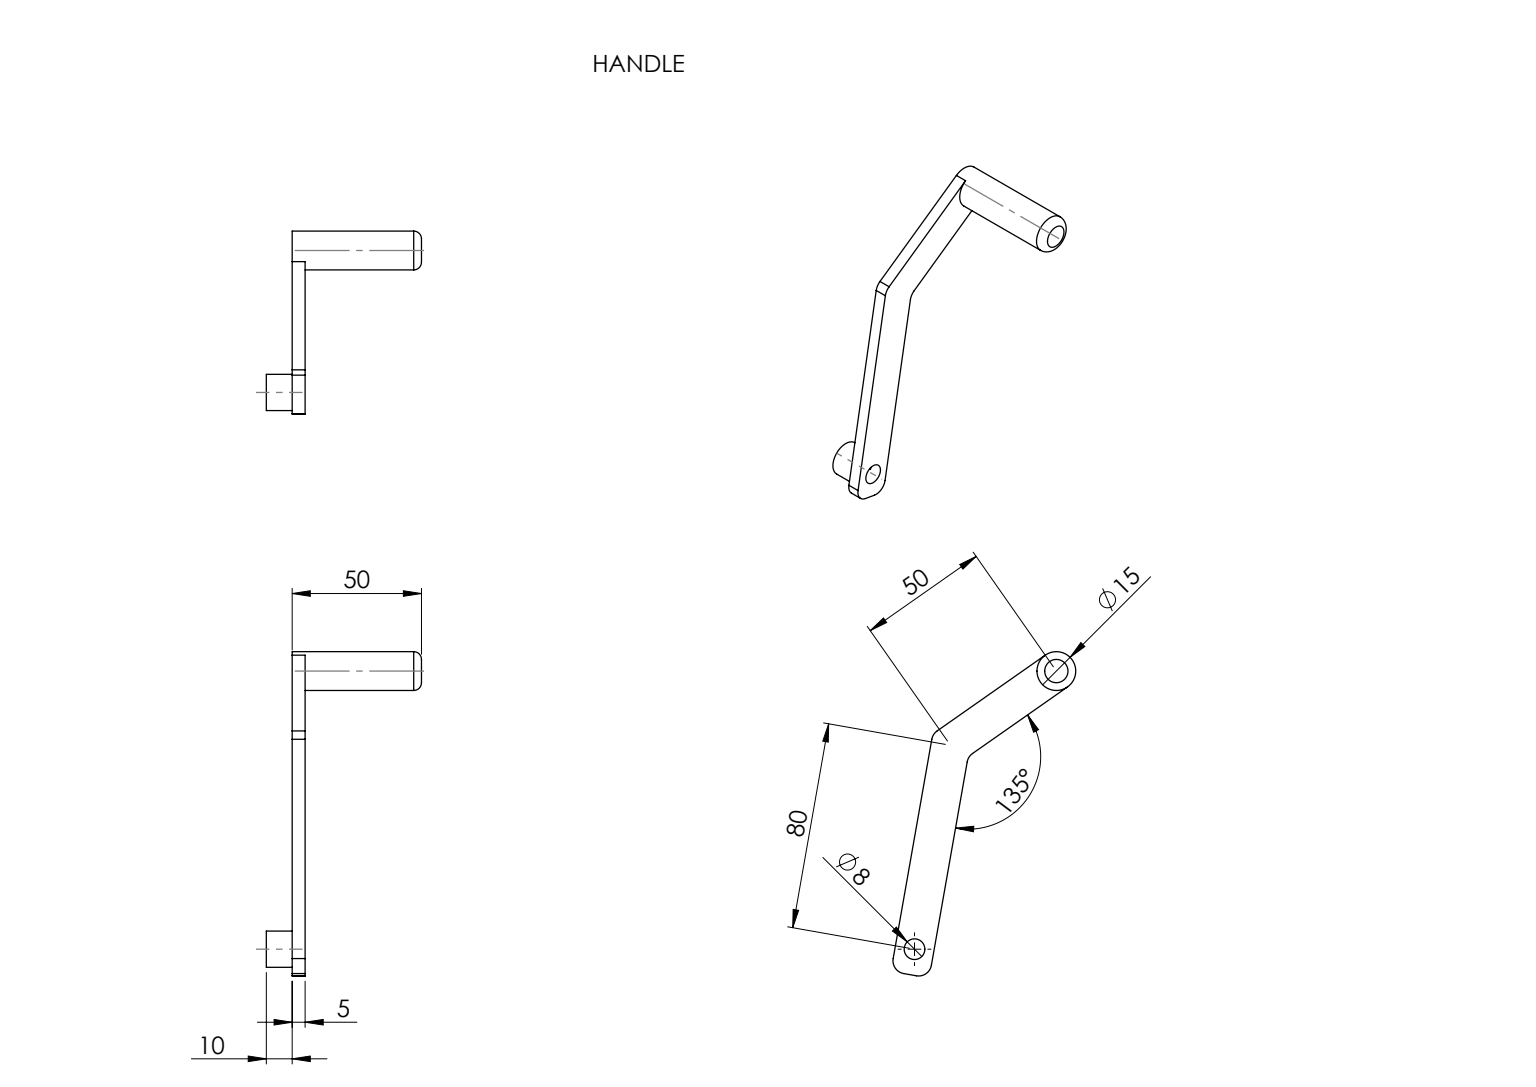
ISO-10303-21;
HEADER;
FILE_DESCRIPTION (('STEP AP214'),
    '1' );
FILE_NAME ('handle.step',
    '2026-09-28T15:49:00',
    ( '' ),
    ( '' ),
    'SwSTEP 2.0',
    'SolidWorks 2026',
    '' );
FILE_SCHEMA (( 'AUTOMOTIVE_DESIGN' ));
ENDSEC;

DATA;
#56=CARTESIAN_POINT ( 'NONE',  ( 55.00000000000000711, -25.98076211353320986, 88.99999999999994316 ) ) ;
#130=ORIENTED_EDGE ( 'NONE', *, *, #26286, .T. ) ;
#133=ORIENTED_EDGE ( 'NONE', *, *, #25065, .T. ) ;
#143=EDGE_CURVE ( 'NONE', #14032, #9695, #27885, .T. ) ;
#156=CARTESIAN_POINT ( 'NONE',  ( 65.00000000000001421, 81.48267994499606459, 30.15054357219658954 ) ) ;
#190=ADVANCED_FACE ( 'NONE', ( #12334 ), #23311, .F. ) ;
#261=AXIS2_PLACEMENT_3D ( 'NONE', #4805, #2292, #35227 ) ;
#346=FILL_AREA_STYLE ('',( #33832 ) ) ;
#366=DIRECTION ( 'NONE',  ( -1.000000000000000000, 0.000000000000000000, 0.000000000000000000 ) ) ;
#383=EDGE_CURVE ( 'NONE', #18596, #21774, #10521, .T. ) ;
#428=VERTEX_POINT ( 'NONE', #27465 ) ;
#447=VECTOR ( 'NONE', #3446, 1000.000000000000000 ) ;
#515=DIRECTION ( 'NONE',  ( 0.000000000000000000, 0.000000000000000000, 1.000000000000000000 ) ) ;
#636=CARTESIAN_POINT ( 'NONE',  ( 70.00000000000001421, -37.13120097615721704, 79.35042362907756797 ) ) ;
#776=CARTESIAN_POINT ( 'NONE',  ( 70.00000000000001421, 87.62632027716348659, 34.45236684482946288 ) ) ;
#781=CARTESIAN_POINT ( 'NONE',  ( 70.00000000000001421, 45.53424681125909501, 59.69714175238111409 ) ) ;
#809=FACE_OUTER_BOUND ( 'NONE', #28343, .T. ) ;
#841=AXIS2_PLACEMENT_3D ( 'NONE', #19896, #5545, #8749 ) ;
#904=EDGE_CURVE ( 'NONE', #3203, #33824, #4242, .T. ) ;
#982=CARTESIAN_POINT ( 'NONE',  ( 65.00000000000001421, -25.98076211353320986, 84.99999999999994316 ) ) ;
#1054=CARTESIAN_POINT ( 'NONE',  ( 70.00000000000001421, -30.47068043442695284, 88.33026027086506815 ) ) ;
#1165=SURFACE_STYLE_FILL_AREA ( #31929 ) ;
#1182=FACE_OUTER_BOUND ( 'NONE', #21588, .T. ) ;
#1194=LINE ( 'NONE', #23141, #2335 ) ;
#1235=CARTESIAN_POINT ( 'NONE',  ( 65.00000000000001421, -25.98076211353320986, 84.99999999999994316 ) ) ;
#1255=DIRECTION ( 'NONE',  ( 1.000000000000000000, -0.000000000000000000, -0.000000000000000000 ) ) ;
#1269=EDGE_LOOP ( 'NONE', ( #4591, #17269, #21862, #33608, #20840, #6158, #6470, #4785 ) ) ;
#1271=ORIENTED_EDGE ( 'NONE', *, *, #26959, .F. ) ;
#1314=DIRECTION ( 'NONE',  ( 0.000000000000000000, -8.326672684688666165E-15, 1.000000000000000000 ) ) ;
#1354=DIRECTION ( 'NONE',  ( 0.000000000000000000, -0.1736481776669211718, -0.9848077530122096857 ) ) ;
#1451=CIRCLE ( 'NONE', #16950, 7.499999999999992895 ) ;
#1492=ORIENTED_EDGE ( 'NONE', *, *, #25065, .F. ) ;
#1496=ORIENTED_EDGE ( 'NONE', *, *, #16220, .F. ) ;
#1573=CARTESIAN_POINT ( 'NONE',  ( 70.00001200000002655, -29.87665282020647695, 83.95300846256282057 ) ) ;
#1611=TOROIDAL_SURFACE ( 'NONE', #5092, 4.499999999999990230, 3.000000000000000000 ) ;
#1670=LINE ( 'NONE', #12654, #13772 ) ;
#1760=CARTESIAN_POINT ( 'NONE',  ( 55.00000000000000711, -26.94801722181409431, 85.25380613764163229 ) ) ;
#1767=LINE ( 'NONE', #20817, #16991 ) ;
#1817=PLANE ( 'NONE',  #32446 ) ;
#1843=EDGE_CURVE ( 'NONE', #25616, #5216, #33585, .T. ) ;
#1888=( NAMED_UNIT ( * ) PLANE_ANGLE_UNIT ( ) SI_UNIT ( $, .RADIAN. ) );
#1954=VERTEX_POINT ( 'NONE', #21205 ) ;
#1975=AXIS2_PLACEMENT_3D ( 'NONE', #6813, #4502, #17962 ) ;
#2064=ADVANCED_FACE ( 'NONE', ( #14500 ), #4316, .T. ) ;
#2150=DIRECTION ( 'NONE',  ( -1.000000000000000000, 0.000000000000000000, 0.000000000000000000 ) ) ;
#2194=ORIENTED_EDGE ( 'NONE', *, *, #3621, .F. ) ;
#2216=ORIENTED_EDGE ( 'NONE', *, *, #904, .F. ) ;
#2232=PLANE ( 'NONE',  #16375 ) ;
#2253=VECTOR ( 'NONE', #6220, 1000.000000000000114 ) ;
#2276=DIRECTION ( 'NONE',  ( 0.000000000000000000, 0.000000000000000000, 1.000000000000000000 ) ) ;
#2292=DIRECTION ( 'NONE',  ( -1.000000000000000000, -0.000000000000000000, -0.000000000000000000 ) ) ;
#2335=VECTOR ( 'NONE', #23318, 999.9999999999998863 ) ;
#2380=CARTESIAN_POINT ( 'NONE',  ( 70.00001200000004076, -24.93377057609608372, 88.89589070667321380 ) ) ;
#2403=DIRECTION ( 'NONE',  ( 0.000000000000000000, -2.775557561562888984E-15, 1.000000000000000000 ) ) ;
#2413=CARTESIAN_POINT ( 'NONE',  ( 65.00000000000001421, -25.98076211353320986, 88.99999999999994316 ) ) ;
#2450=ADVANCED_FACE ( 'NONE', ( #15932 ), #18461, .T. ) ;
#2497=CARTESIAN_POINT ( 'NONE',  ( 70.00000000000001421, -29.60243954609234507, 93.25429903592612391 ) ) ;
#2565=VERTEX_POINT ( 'NONE', #27993 ) ;
#2569=CARTESIAN_POINT ( 'NONE',  ( 65.00000000000001421, 75.33903961282865680, 25.84872029956372330 ) ) ;
#2593=ORIENTED_EDGE ( 'NONE', *, *, #13307, .T. ) ;
#2628=LINE ( 'NONE', #10536, #17242 ) ;
#2636=CYLINDRICAL_SURFACE ( 'NONE', #35102, 5.000000000000004441 ) ;
#2663=EDGE_CURVE ( 'NONE', #3203, #18596, #9362, .T. ) ;
#2735=DIRECTION ( 'NONE',  ( 0.000000000000000000, 0.000000000000000000, -1.000000000000000000 ) ) ;
#2741=AXIS2_PLACEMENT_3D ( 'NONE', #19253, #30776, #2735 ) ;
#2745=ORIENTED_EDGE ( 'NONE', *, *, #4160, .F. ) ;
#2809=CARTESIAN_POINT ( 'NONE',  ( 65.00000000000001421, 87.62632027716348659, 34.45236684482946288 ) ) ;
#2854=VERTEX_POINT ( 'NONE', #6203 ) ;
#2954=EDGE_CURVE ( 'NONE', #9823, #7205, #23657, .T. ) ;
#3203=VERTEX_POINT ( 'NONE', #10117 ) ;
#3222=CARTESIAN_POINT ( 'NONE',  ( 65.00000000000001421, -30.47068043442695284, 88.33026027086506815 ) ) ;
#3229=CARTESIAN_POINT ( 'NONE',  ( 65.00000000000001421, -32.20716221109618260, 78.48218274074299927 ) ) ;
#3232=AXIS2_PLACEMENT_3D ( 'NONE', #781, #25461, #19843 ) ;
#3269=DIRECTION ( 'NONE',  ( 0.000000000000000000, 0.2538061376417697357, 0.9672551082808334977 ) ) ;
#3276=ORIENTED_EDGE ( 'NONE', *, *, #9282, .T. ) ;
#3368=DIRECTION ( 'NONE',  ( 0.000000000000000000, 0.000000000000000000, 1.000000000000000000 ) ) ;
#3388=ORIENTED_EDGE ( 'NONE', *, *, #16220, .T. ) ;
#3389=EDGE_CURVE ( 'NONE', #2565, #13276, #17096, .T. ) ;
#3416=EDGE_CURVE ( 'NONE', #33336, #30332, #7608, .T. ) ;
#3446=DIRECTION ( 'NONE',  ( 1.000000000000000000, -0.000000000000000000, -0.000000000000000000 ) ) ;
#3489=CARTESIAN_POINT ( 'NONE',  ( 65.00000000000001421, -25.98076211353320986, 80.99999999999992895 ) ) ;
#3511=DIRECTION ( 'NONE',  ( 0.000000000000000000, 0.000000000000000000, 1.000000000000000000 ) ) ;
#3621=EDGE_CURVE ( 'NONE', #4878, #28758, #31678, .T. ) ;
#3638=ORIENTED_EDGE ( 'NONE', *, *, #5358, .T. ) ;
#3683=CARTESIAN_POINT ( 'NONE',  ( 70.00000000000001421, 0.000000000000000000, 0.000000000000000000 ) ) ;
#3724=ORIENTED_EDGE ( 'NONE', *, *, #24002, .T. ) ;
#3746=CIRCLE ( 'NONE', #17524, 5.000000000000004441 ) ;
#3769=CLOSED_SHELL ( 'NONE', ( #18687, #5338, #22527, #33299, #32877, #34808, #14774, #29471, #2450, #190, #15138, #32497, #4472, #4930, #4111, #33091, #6476, #7953, #7065, #31290, #10902, #2064, #24425, #21358, #22284, #3966 ) ) ;
#3787=ORIENTED_EDGE ( 'NONE', *, *, #14974, .T. ) ;
#3796=CARTESIAN_POINT ( 'NONE',  ( 112.0000000000000000, 81.48267994499606459, 37.65054357219658243 ) ) ;
#3860=CARTESIAN_POINT ( 'NONE',  ( 70.00000000000001421, -30.47068043442695284, 93.33026027086508236 ) ) ;
#3893=PLANE ( 'NONE',  #22062 ) ;
#3910=VECTOR ( 'NONE', #4653, 999.9999999999998863 ) ;
#3932=CARTESIAN_POINT ( 'NONE',  ( 70.00001200000002655, -29.17942948312593998, 82.54181312010028648 ) ) ;
#3966=ADVANCED_FACE ( 'NONE', ( #5911 ), #17055, .F. ) ;
#3993=EDGE_CURVE ( 'NONE', #20175, #14032, #8812, .T. ) ;
#4111=ADVANCED_FACE ( 'NONE', ( #25901, #17767 ), #23356, .T. ) ;
#4136=( NAMED_UNIT ( * ) SI_UNIT ( $, .STERADIAN. ) SOLID_ANGLE_UNIT ( ) );
#4160=EDGE_CURVE ( 'NONE', #34443, #26484, #18590, .T. ) ;
#4235=ORIENTED_EDGE ( 'NONE', *, *, #8593, .T. ) ;
#4241=DIRECTION ( 'NONE',  ( 0.000000000000000000, 0.000000000000000000, 1.000000000000000000 ) ) ;
#4242=CIRCLE ( 'NONE', #30675, 4.499999999999990230 ) ;
#4271=EDGE_CURVE ( 'NONE', #2854, #9753, #31822, .T. ) ;
#4316=TOROIDAL_SURFACE ( 'NONE', #841, 4.499999999999990230, 3.000000000000000000 ) ;
#4373=ORIENTED_EDGE ( 'NONE', *, *, #3621, .T. ) ;
#4472=ADVANCED_FACE ( 'NONE', ( #809 ), #3893, .T. ) ;
#4502=DIRECTION ( 'NONE',  ( -1.000000000000000000, 0.000000000000000000, 0.000000000000000000 ) ) ;
#4503=ORIENTED_EDGE ( 'NONE', *, *, #17218, .F. ) ;
#4521=STYLED_ITEM ( 'NONE', ( #15434 ), #33750 ) ;
#4547=SHAPE_REPRESENTATION ( 'handle', ( #21307 ), #23057 ) ;
#4565=ORIENTED_EDGE ( 'NONE', *, *, #18024, .T. ) ;
#4591=ORIENTED_EDGE ( 'NONE', *, *, #12276, .T. ) ;
#4592=ORIENTED_EDGE ( 'NONE', *, *, #3389, .T. ) ;
#4617=DIRECTION ( 'NONE',  ( -0.000000000000000000, 0.8191520442889889120, 0.5735764363510502672 ) ) ;
#4632=ORIENTED_EDGE ( 'NONE', *, *, #7310, .T. ) ;
#4653=DIRECTION ( 'NONE',  ( 0.000000000000000000, 0.5735764363510502672, -0.8191520442889889120 ) ) ;
#4693=CYLINDRICAL_SURFACE ( 'NONE', #5183, 4.000000000000003553 ) ;
#4695=MECHANICAL_DESIGN_GEOMETRIC_PRESENTATION_REPRESENTATION('',(#10435),#28238);
#4730=CARTESIAN_POINT ( 'NONE',  ( 70.00000600000001327, -25.98076211353320986, 88.99999999999994316 ) ) ;
#4785=ORIENTED_EDGE ( 'NONE', *, *, #14974, .F. ) ;
#4805=CARTESIAN_POINT ( 'NONE',  ( 65.00000000000001421, -25.98076211353320986, 84.99999999999994316 ) ) ;
#4816=ORIENTED_EDGE ( 'NONE', *, *, #1843, .T. ) ;
#4878=VERTEX_POINT ( 'NONE', #31685 ) ;
#4930=ADVANCED_FACE ( 'NONE', ( #14936 ), #1817, .F. ) ;
#4995=FACE_OUTER_BOUND ( 'NONE', #23443, .T. ) ;
#5038=DIRECTION ( 'NONE',  ( 1.000000000000000000, -0.000000000000000000, -0.000000000000000000 ) ) ;
#5075=CARTESIAN_POINT ( 'NONE',  ( 65.00000000000001421, -30.47068043442695284, 93.33026027086508236 ) ) ;
#5076=VERTEX_POINT ( 'NONE', #32578 ) ;
#5078=CARTESIAN_POINT ( 'NONE',  ( 70.00001200000002655, -22.78209474394049039, 87.45818687989959983 ) ) ;
#5092=AXIS2_PLACEMENT_3D ( 'NONE', #30970, #366, #22858 ) ;
#5114=DIRECTION ( 'NONE',  ( -1.000000000000000000, -0.000000000000000000, -0.000000000000000000 ) ) ;
#5183=AXIS2_PLACEMENT_3D ( 'NONE', #18695, #7891, #21221 ) ;
#5209=EDGE_LOOP ( 'NONE', ( #23961, #2216, #35094, #7402 ) ) ;
#5216=VERTEX_POINT ( 'NONE', #33292 ) ;
#5272=CARTESIAN_POINT ( 'NONE',  ( 65.00000000000001421, -30.47068043442695284, 88.33026027086506815 ) ) ;
#5338=ADVANCED_FACE ( 'NONE', ( #22118 ), #5580, .T. ) ;
#5358=EDGE_CURVE ( 'NONE', #9823, #30224, #18658, .T. ) ;
#5379=AXIS2_PLACEMENT_3D ( 'NONE', #24595, #35586, #16814 ) ;
#5388=CARTESIAN_POINT ( 'NONE',  ( 55.00000000000000711, -25.99649394950422021, 81.00003093645240426 ) ) ;
#5395=AXIS2_PLACEMENT_3D ( 'NONE', #13673, #8252, #25002 ) ;
#5424=ORIENTED_EDGE ( 'NONE', *, *, #18024, .F. ) ;
#5445=DIRECTION ( 'NONE',  ( 1.000000000000000000, -0.000000000000000000, -0.000000000000000000 ) ) ;
#5473=PLANE ( 'NONE',  #10506 ) ;
#5484=ORIENTED_EDGE ( 'NONE', *, *, #20613, .F. ) ;
#5509=AXIS2_PLACEMENT_3D ( 'NONE', #21410, #7726, #18709 ) ;
#5515=EDGE_LOOP ( 'NONE', ( #12905, #15381 ) ) ;
#5545=DIRECTION ( 'NONE',  ( -1.000000000000000000, 0.000000000000000000, 0.000000000000000000 ) ) ;
#5580=CYLINDRICAL_SURFACE ( 'NONE', #27312, 7.499999999999992895 ) ;
#5598=DIRECTION ( 'NONE',  ( -1.000000000000000000, 0.000000000000000000, 0.000000000000000000 ) ) ;
#5723=EDGE_CURVE ( 'NONE', #25950, #34599, #1451, .T. ) ;
#5787=CARTESIAN_POINT ( 'NONE',  ( 55.00000000000000711, -25.98076211353320986, 84.99999999999994316 ) ) ;
#5849=ORIENTED_EDGE ( 'NONE', *, *, #14083, .T. ) ;
#5911=FACE_OUTER_BOUND ( 'NONE', #7615, .T. ) ;
#5954=LINE ( 'NONE', #25404, #447 ) ;
#5971=ORIENTED_EDGE ( 'NONE', *, *, #4271, .F. ) ;
#6022=ORIENTED_EDGE ( 'NONE', *, *, #14553, .F. ) ;
#6025=CARTESIAN_POINT ( 'NONE',  ( 55.00000000000000711, -25.98076211353320986, 80.99999999999992895 ) ) ;
#6145=ORIENTED_EDGE ( 'NONE', *, *, #14083, .F. ) ;
#6148=VECTOR ( 'NONE', #16787, 1000.000000000000000 ) ;
#6158=ORIENTED_EDGE ( 'NONE', *, *, #10194, .T. ) ;
#6159=ORIENTED_EDGE ( 'NONE', *, *, #3389, .F. ) ;
#6192=DIRECTION ( 'NONE',  ( -1.000000000000000000, 0.000000000000000000, 0.000000000000000000 ) ) ;
#6203=CARTESIAN_POINT ( 'NONE',  ( 65.00000000000001421, 49.63000703270403591, 62.56502393413636298 ) ) ;
#6220=DIRECTION ( 'NONE',  ( 0.000000000000000000, -0.2538061376417682924, -0.9672551082808338307 ) ) ;
#6295=ORIENTED_EDGE ( 'NONE', *, *, #26286, .F. ) ;
#6385=COLOUR_RGB ( '', 0.08235294, 0.09019608, 0.10196078) ;
#6409=AXIS2_PLACEMENT_3D ( 'NONE', #7493, #29294, #29648 ) ;
#6470=ORIENTED_EDGE ( 'NONE', *, *, #15880, .F. ) ;
#6472=CARTESIAN_POINT ( 'NONE',  ( 70.00000000000001421, -24.67840078103129997, 92.38605814759151258 ) ) ;
#6476=ADVANCED_FACE ( 'NONE', ( #28695 ), #28867, .F. ) ;
#6496=VECTOR ( 'NONE', #6192, 1000.000000000000000 ) ;
#6530=DIRECTION ( 'NONE',  ( -1.000000000000000000, -0.000000000000000000, -0.000000000000000000 ) ) ;
#6553=CARTESIAN_POINT ( 'NONE',  ( 70.00000000000001421, 58.35354061212520804, 76.25822877525452270 ) ) ;
#6707=CARTESIAN_POINT ( 'NONE',  ( 112.0000000000000000, 81.48267994499606459, 22.65054357219659664 ) ) ;
#6723=DIRECTION ( 'NONE',  ( -1.000000000000000000, 0.000000000000000000, 0.000000000000000000 ) ) ;
#6813=CARTESIAN_POINT ( 'NONE',  ( 70.00000000000001421, 45.53424681125909501, 59.69714175238111409 ) ) ;
#6927=DIRECTION ( 'NONE',  ( 0.000000000000000000, 0.9672551082808338307, -0.2538061376417690695 ) ) ;
#6962=CARTESIAN_POINT ( 'NONE',  ( 70.00001200000002655, -27.02775365097034310, 88.89589070667321380 ) ) ;
#6974=AXIS2_PLACEMENT_3D ( 'NONE', #21555, #34927, #10253 ) ;
#7016=DIRECTION ( 'NONE',  ( -0.000000000000000000, 0.2538061376417689585, 0.9672551082808338307 ) ) ;
#7063=VECTOR ( 'NONE', #16180, 1000.000000000000114 ) ;
#7065=ADVANCED_FACE ( 'NONE', ( #24276 ), #18186, .T. ) ;
#7102=CARTESIAN_POINT ( 'NONE',  ( 63.00000000000001421, -26.94801722181409431, 85.25380613764163229 ) ) ;
#7166=( LENGTH_UNIT ( ) NAMED_UNIT ( * ) SI_UNIT ( .MILLI., .METRE. ) );
#7205=VERTEX_POINT ( 'NONE', #21910 ) ;
#7282=DIRECTION ( 'NONE',  ( 0.000000000000000000, 0.2538061376417690140, 0.9672551082808337197 ) ) ;
#7310=EDGE_CURVE ( 'NONE', #428, #2565, #16848, .T. ) ;
#7388=ORIENTED_EDGE ( 'NONE', *, *, #28035, .F. ) ;
#7402=ORIENTED_EDGE ( 'NONE', *, *, #31805, .F. ) ;
#7466=CARTESIAN_POINT ( 'NONE',  ( 115.0000000000000000, 81.48267994499606459, 37.65054357219658243 ) ) ;
#7484=ORIENTED_EDGE ( 'NONE', *, *, #24002, .F. ) ;
#7493=CARTESIAN_POINT ( 'NONE',  ( 112.0000000000000000, 81.48267994499606459, 30.15054357219658954 ) ) ;
#7563=CARTESIAN_POINT ( 'NONE',  ( 70.00000000000001421, -35.39471919948800149, 89.19850115919967948 ) ) ;
#7576=CARTESIAN_POINT ( 'NONE',  ( 70.00001200000001234, -25.45716333793490449, 88.99999999999995737 ) ) ;
#7608=CIRCLE ( 'NONE', #27751, 4.000000000000003553 ) ;
#7615=EDGE_LOOP ( 'NONE', ( #33702, #6159, #32414, #32946 ) ) ;
#7645=CARTESIAN_POINT ( 'NONE',  ( 55.00000000000000711, -25.98076211353320986, 91.99999999999994316 ) ) ;
#7662=AXIS2_PLACEMENT_3D ( 'NONE', #1054, #12025, #28593 ) ;
#7714=EDGE_CURVE ( 'NONE', #28924, #33336, #16617, .T. ) ;
#7726=DIRECTION ( 'NONE',  ( 1.000000000000000000, 0.000000000000000000, 0.000000000000000000 ) ) ;
#7891=DIRECTION ( 'NONE',  ( -1.000000000000000000, -0.000000000000000000, -0.000000000000000000 ) ) ;
#7953=ADVANCED_FACE ( 'NONE', ( #4995 ), #32519, .T. ) ;
#7969=CARTESIAN_POINT ( 'NONE',  ( 65.00000000000001421, -25.98076211353320986, 84.99999999999994316 ) ) ;
#7971=ORIENTED_EDGE ( 'NONE', *, *, #8556, .F. ) ;
#8023=APPLICATION_CONTEXT ( 'automotive_design' ) ;
#8024=VECTOR ( 'NONE', #27137, 1000.000000000000000 ) ;
#8070=CARTESIAN_POINT ( 'NONE',  ( 115.0000000000000000, 81.48267994499606459, 30.15054357219658954 ) ) ;
#8101=ORIENTED_EDGE ( 'NONE', *, *, #10457, .T. ) ;
#8185=ORIENTED_EDGE ( 'NONE', *, *, #8641, .F. ) ;
#8187=CARTESIAN_POINT ( 'NONE',  ( 70.00000000000001421, -30.47068043442695284, 93.33026027086508236 ) ) ;
#8219=CIRCLE ( 'NONE', #32956, 2.999999999999999112 ) ;
#8231=AXIS2_PLACEMENT_3D ( 'NONE', #20104, #34354, #28769 ) ;
#8236=DIRECTION ( 'NONE',  ( -1.000000000000000000, 0.000000000000000000, 0.000000000000000000 ) ) ;
#8252=DIRECTION ( 'NONE',  ( 1.000000000000000000, 0.000000000000000000, 0.000000000000000000 ) ) ;
#8387=CARTESIAN_POINT ( 'NONE',  ( 115.0000000000000000, 81.48267994499606459, 22.65054357219660019 ) ) ;
#8498=APPLICATION_CONTEXT ( 'automotive_design' ) ;
#8556=EDGE_CURVE ( 'NONE', #22699, #26100, #14156, .T. ) ;
#8577=ORIENTED_EDGE ( 'NONE', *, *, #13892, .F. ) ;
#8593=EDGE_CURVE ( 'NONE', #26100, #18471, #30872, .T. ) ;
#8598=DIRECTION ( 'NONE',  ( -1.000000000000000000, 0.000000000000000000, 0.000000000000000000 ) ) ;
#8641=EDGE_CURVE ( 'NONE', #30224, #9823, #29729, .T. ) ;
#8657=AXIS2_PLACEMENT_3D ( 'NONE', #3222, #8598, #31108 ) ;
#8749=DIRECTION ( 'NONE',  ( 0.000000000000000000, 0.000000000000000000, 1.000000000000000000 ) ) ;
#8758=CIRCLE ( 'NONE', #31187, 7.000000000000006217 ) ;
#8783=ORIENTED_EDGE ( 'NONE', *, *, #32390, .T. ) ;
#8812=CIRCLE ( 'NONE', #25512, 5.000000000000004441 ) ;
#8843=DIRECTION ( 'NONE',  ( 0.000000000000000000, -0.5735764363510502672, 0.8191520442889889120 ) ) ;
#8939=VECTOR ( 'NONE', #24663, 1000.000000000000000 ) ;
#8980=ORIENTED_EDGE ( 'NONE', *, *, #15855, .T. ) ;
#8999=FACE_OUTER_BOUND ( 'NONE', #35131, .T. ) ;
#9112=ORIENTED_EDGE ( 'NONE', *, *, #25441, .F. ) ;
#9282=EDGE_CURVE ( 'NONE', #28214, #20788, #9990, .T. ) ;
#9284=CARTESIAN_POINT ( 'NONE',  ( 70.00000000000001421, 75.33903961282865680, 25.84872029956372685 ) ) ;
#9308=PRODUCT_CONTEXT ( 'NONE', #8023, 'mechanical' ) ;
#9336=ORIENTED_EDGE ( 'NONE', *, *, #21823, .F. ) ;
#9362=CIRCLE ( 'NONE', #5379, 3.000000000000002665 ) ;
#9541=EDGE_CURVE ( 'NONE', #5076, #22699, #25456, .T. ) ;
#9617=( NAMED_UNIT ( * ) SI_UNIT ( $, .STERADIAN. ) SOLID_ANGLE_UNIT ( ) );
#9670=CARTESIAN_POINT ( 'NONE',  ( 70.00000600000001327, -25.98076211353320986, 80.99999999999992895 ) ) ;
#9695=VERTEX_POINT ( 'NONE', #23821 ) ;
#9753=VERTEX_POINT ( 'NONE', #17690 ) ;
#9793=PRESENTATION_STYLE_ASSIGNMENT (( #20930 ) ) ;
#9823=VERTEX_POINT ( 'NONE', #16588 ) ;
#9827=EDGE_LOOP ( 'NONE', ( #22446, #8185, #12994, #133 ) ) ;
#9839=CARTESIAN_POINT ( 'NONE',  ( 70.00001200000001234, -28.43894899343287364, 81.80133263040721658 ) ) ;
#9939=EDGE_CURVE ( 'NONE', #13682, #34443, #16635, .T. ) ;
#9948=EDGE_CURVE ( 'NONE', #14032, #25616, #30106, .T. ) ;
#9955=VECTOR ( 'NONE', #17634, 1000.000000000000114 ) ;
#9990=LINE ( 'NONE', #20951, #12497 ) ;
#10033=LINE ( 'NONE', #1760, #17459 ) ;
#10043=CARTESIAN_POINT ( 'NONE',  ( 65.00000000000001421, 54.25778039068027425, 73.39034659349927381 ) ) ;
#10051=ORIENTED_EDGE ( 'NONE', *, *, #2954, .T. ) ;
#10117=CARTESIAN_POINT ( 'NONE',  ( 115.0000000000000000, 81.48267994499606459, 34.65054357219658243 ) ) ;
#10158=DIRECTION ( 'NONE',  ( 0.000000000000000000, 0.000000000000000000, -1.000000000000000000 ) ) ;
#10169=VECTOR ( 'NONE', #16839, 1000.000000000000000 ) ;
#10180=CARTESIAN_POINT ( 'NONE',  ( 65.00000000000001421, 81.48267994499606459, 22.65054357219659664 ) ) ;
#10194=EDGE_CURVE ( 'NONE', #33932, #1954, #10580, .T. ) ;
#10253=DIRECTION ( 'NONE',  ( 0.000000000000000000, 0.000000000000000000, 1.000000000000000000 ) ) ;
#10357=DIRECTION ( 'NONE',  ( 0.000000000000000000, 0.9848077530122095746, -0.1736481776669212829 ) ) ;
#10383=ORIENTED_EDGE ( 'NONE', *, *, #10194, .F. ) ;
#10385=ADVANCED_BREP_SHAPE_REPRESENTATION ( '', ( #33750, #21307 ), #23057 ) ;
#10435=STYLED_ITEM ( 'NONE', ( #9793 ), #10385 ) ;
#10457=EDGE_CURVE ( 'NONE', #5216, #25950, #1194, .T. ) ;
#10469=ORIENTED_EDGE ( 'NONE', *, *, #18244, .T. ) ;
#10506=AXIS2_PLACEMENT_3D ( 'NONE', #6472, #25400, #25576 ) ;
#10521=CIRCLE ( 'NONE', #11666, 7.499999999999992895 ) ;
#10536=CARTESIAN_POINT ( 'NONE',  ( 70.00000000000001421, 58.94749845961094792, 75.40996905927893579 ) ) ;
#10580=LINE ( 'NONE', #12928, #18928 ) ;
#10625=EDGE_LOOP ( 'NONE', ( #8101, #26620, #15965, #25478, #32511, #9112, #26990, #33425, #7388, #30388, #31670, #4816 ) ) ;
#10766=AXIS2_PLACEMENT_3D ( 'NONE', #28124, #30645, #8843 ) ;
#10829=EDGE_CURVE ( 'NONE', #16551, #5076, #2628, .T. ) ;
#10830=MECHANICAL_DESIGN_GEOMETRIC_PRESENTATION_REPRESENTATION('',(#4521),#13125);
#10856=ORIENTED_EDGE ( 'NONE', *, *, #24635, .T. ) ;
#10902=ADVANCED_FACE ( 'NONE', ( #19673 ), #30687, .F. ) ;
#10933=CARTESIAN_POINT ( 'NONE',  ( 65.00000000000001421, -25.99649394950422021, 81.00003093645240426 ) ) ;
#10970=DIRECTION ( 'NONE',  ( 1.000000000000000000, -0.000000000000000000, -0.000000000000000000 ) ) ;
#11081=ORIENTED_EDGE ( 'NONE', *, *, #10457, .F. ) ;
#11133=ORIENTED_EDGE ( 'NONE', *, *, #22650, .T. ) ;
#11166=FACE_OUTER_BOUND ( 'NONE', #17342, .T. ) ;
#11238=LINE ( 'NONE', #3860, #6496 ) ;
#11272=DIRECTION ( 'NONE',  ( 1.000000000000000000, -0.000000000000000000, -0.000000000000000000 ) ) ;
#11318=AXIS2_PLACEMENT_3D ( 'NONE', #35262, #29197, #31872 ) ;
#11357=AXIS2_PLACEMENT_3D ( 'NONE', #12990, #26509, #27215 ) ;
#11421=DIRECTION ( 'NONE',  ( 0.000000000000000000, 0.000000000000000000, 1.000000000000000000 ) ) ;
#11545=CIRCLE ( 'NONE', #8657, 5.000000000000004441 ) ;
#11556=PLANE ( 'NONE',  #10766 ) ;
#11601=( NAMED_UNIT ( * ) SI_UNIT ( $, .STERADIAN. ) SOLID_ANGLE_UNIT ( ) );
#11666=AXIS2_PLACEMENT_3D ( 'NONE', #29808, #24579, #2276 ) ;
#11683=CARTESIAN_POINT ( 'NONE',  ( 70.00000000000001421, -35.39471919948800149, 89.19850115919967948 ) ) ;
#11826=DIRECTION ( 'NONE',  ( 0.000000000000000000, 0.5735764363510502672, -0.8191520442889889120 ) ) ;
#11961=DIRECTION ( 'NONE',  ( -1.000000000000000000, -0.000000000000000000, -0.000000000000000000 ) ) ;
#12025=DIRECTION ( 'NONE',  ( 1.000000000000000000, -0.000000000000000000, -0.000000000000000000 ) ) ;
#12032=CARTESIAN_POINT ( 'NONE',  ( 65.00000000000001421, -29.60243954609234507, 93.25429903592612391 ) ) ;
#12139=SHAPE_REPRESENTATION_RELATIONSHIP ( 'NONE' , 'NONE' ,  #4547, #10385 ) ;
#12276=EDGE_CURVE ( 'NONE', #28609, #28924, #25007, .T. ) ;
#12331=ORIENTED_EDGE ( 'NONE', *, *, #383, .F. ) ;
#12334=FACE_OUTER_BOUND ( 'NONE', #27825, .T. ) ;
#12437=EDGE_LOOP ( 'NONE', ( #27860, #32855, #3787, #16372 ) ) ;
#12463=EDGE_LOOP ( 'NONE', ( #25660, #3638 ) ) ;
#12497=VECTOR ( 'NONE', #10357, 1000.000000000000114 ) ;
#12553=CARTESIAN_POINT ( 'NONE',  ( 70.00000600000001327, -25.98076211353320986, 88.99999999999994316 ) ) ;
#12616=DIRECTION ( 'NONE',  ( 0.000000000000000000, -0.9848077530122092416, 0.1736481776669233923 ) ) ;
#12654=CARTESIAN_POINT ( 'NONE',  ( 65.00000000000001421, -27.28312344603513040, 77.61394185240837373 ) ) ;
#12676=FACE_BOUND ( 'NONE', #5515, .T. ) ;
#12697=PRODUCT_DEFINITION_SHAPE ( 'NONE', 'NONE',  #22682 ) ;
#12725=DIRECTION ( 'NONE',  ( 0.000000000000000000, 0.000000000000000000, 1.000000000000000000 ) ) ;
#12768=AXIS2_PLACEMENT_3D ( 'NONE', #15013, #14841, #4241 ) ;
#12800=DIRECTION ( 'NONE',  ( 0.000000000000000000, 0.000000000000000000, 1.000000000000000000 ) ) ;
#12858=EDGE_LOOP ( 'NONE', ( #34913, #10051, #8783, #9336 ) ) ;
#12872=CARTESIAN_POINT ( 'NONE',  ( 70.00000000000001421, -36.26296008782259861, 84.27446239413865214 ) ) ;
#12905=ORIENTED_EDGE ( 'NONE', *, *, #12276, .F. ) ;
#12928=CARTESIAN_POINT ( 'NONE',  ( 75.00000000000002842, -27.93100416606587899, 81.50764321173589622 ) ) ;
#12990=CARTESIAN_POINT ( 'NONE',  ( 55.00000000000000711, -25.98076211353320986, 84.99999999999994316 ) ) ;
#12994=ORIENTED_EDGE ( 'NONE', *, *, #21823, .T. ) ;
#13000=ORIENTED_EDGE ( 'NONE', *, *, #32390, .F. ) ;
#13004=VECTOR ( 'NONE', #30728, 1000.000000000000000 ) ;
#13021=DIRECTION ( 'NONE',  ( 0.000000000000000000, 0.000000000000000000, 1.000000000000000000 ) ) ;
#13034=CARTESIAN_POINT ( 'NONE',  ( 65.00000000000001421, -25.98076211353320986, 77.99999999999992895 ) ) ;
#13044=ORIENTED_EDGE ( 'NONE', *, *, #32640, .F. ) ;
#13059=AXIS2_PLACEMENT_3D ( 'NONE', #34408, #7016, #34039 ) ;
#13090=VECTOR ( 'NONE', #33810, 1000.000000000000000 ) ;
#13098=VECTOR ( 'NONE', #27328, 1000.000000000000000 ) ;
#13125=( GEOMETRIC_REPRESENTATION_CONTEXT ( 3 ) GLOBAL_UNCERTAINTY_ASSIGNED_CONTEXT ( ( #25139 ) ) GLOBAL_UNIT_ASSIGNED_CONTEXT ( ( #7166, #20654, #4136 ) ) REPRESENTATION_CONTEXT ( 'NONE', 'WORKASPACE' ) );
#13180=CARTESIAN_POINT ( 'NONE',  ( 70.00001200000002655, -25.45716333793490094, 80.99999999999991473 ) ) ;
#13213=DIRECTION ( 'NONE',  ( -1.000000000000000000, -0.000000000000000000, -0.000000000000000000 ) ) ;
#13256=ORIENTED_EDGE ( 'NONE', *, *, #10829, .T. ) ;
#13276=VERTEX_POINT ( 'NONE', #10933 ) ;
#13280=DIRECTION ( 'NONE',  ( 0.000000000000000000, 0.000000000000000000, -1.000000000000000000 ) ) ;
#13307=EDGE_CURVE ( 'NONE', #21774, #26100, #16303, .T. ) ;
#13330=ORIENTED_EDGE ( 'NONE', *, *, #383, .T. ) ;
#13521=ORIENTED_EDGE ( 'NONE', *, *, #18595, .F. ) ;
#13523=CARTESIAN_POINT ( 'NONE',  ( 70.00001200000001234, -23.96628619204960486, 81.50485444658289680 ) ) ;
#13619=AXIS2_PLACEMENT_3D ( 'NONE', #7969, #13213, #23832 ) ;
#13666=ORIENTED_EDGE ( 'NONE', *, *, #29434, .T. ) ;
#13673=CARTESIAN_POINT ( 'NONE',  ( 65.00000000000001421, -25.98076211353320986, 84.99999999999994316 ) ) ;
#13682=VERTEX_POINT ( 'NONE', #18985 ) ;
#13728=CARTESIAN_POINT ( 'NONE',  ( 70.00000000000001421, -27.28312344603513040, 77.61394185240837373 ) ) ;
#13750=ORIENTED_EDGE ( 'NONE', *, *, #24635, .F. ) ;
#13772=VECTOR ( 'NONE', #26148, 1000.000000000000114 ) ;
#13797=CARTESIAN_POINT ( 'NONE',  ( 65.00000000000001421, -25.98076211353320986, 84.99999999999994316 ) ) ;
#13802=CARTESIAN_POINT ( 'NONE',  ( 65.00000000000001421, 45.53424681125909501, 59.69714175238111409 ) ) ;
#13807=DIRECTION ( 'NONE',  ( 0.000000000000000000, 0.000000000000000000, 1.000000000000000000 ) ) ;
#13824=AXIS2_PLACEMENT_3D ( 'NONE', #33554, #31386, #11421 ) ;
#13892=EDGE_CURVE ( 'NONE', #28214, #13682, #18671, .T. ) ;
#13948=DIRECTION ( 'NONE',  ( 0.000000000000000000, 0.1736481776669211718, 0.9848077530122096857 ) ) ;
#14002=CARTESIAN_POINT ( 'NONE',  ( 70.00000000000001421, 75.33903961282864259, 25.84872029956371975 ) ) ;
#14032=VERTEX_POINT ( 'NONE', #28034 ) ;
#14056=ORIENTED_EDGE ( 'NONE', *, *, #33047, .F. ) ;
#14083=EDGE_CURVE ( 'NONE', #5216, #2854, #16849, .T. ) ;
#14156=CIRCLE ( 'NONE', #24533, 7.499999999999992895 ) ;
#14179=DIRECTION ( 'NONE',  ( -1.000000000000000000, -0.000000000000000000, -0.000000000000000000 ) ) ;
#14299=( NAMED_UNIT ( * ) PLANE_ANGLE_UNIT ( ) SI_UNIT ( $, .RADIAN. ) );
#14334=VERTEX_POINT ( 'NONE', #7645 ) ;
#14339=VECTOR ( 'NONE', #29934, 1000.000000000000114 ) ;
#14357=CARTESIAN_POINT ( 'NONE',  ( 70.00000000000001421, -31.33892132276156062, 83.40622150580404082 ) ) ;
#14486=CYLINDRICAL_SURFACE ( 'NONE', #30666, 5.000000000000004441 ) ;
#14500=FACE_OUTER_BOUND ( 'NONE', #5209, .T. ) ;
#14553=EDGE_CURVE ( 'NONE', #32501, #35307, #19512, .T. ) ;
#14559=AXIS2_PLACEMENT_3D ( 'NONE', #13802, #11272, #24790 ) ;
#14562=FACE_OUTER_BOUND ( 'NONE', #21463, .T. ) ;
#14573=FACE_OUTER_BOUND ( 'NONE', #19757, .T. ) ;
#14733=ORIENTED_EDGE ( 'NONE', *, *, #3416, .T. ) ;
#14774=ADVANCED_FACE ( 'NONE', ( #31389, #12676 ), #22923, .F. ) ;
#14838=AXIS2_PLACEMENT_3D ( 'NONE', #16423, #27260, #17931 ) ;
#14841=DIRECTION ( 'NONE',  ( -1.000000000000000000, 0.000000000000000000, 0.000000000000000000 ) ) ;
#14871=ORIENTED_EDGE ( 'NONE', *, *, #33047, .T. ) ;
#14894=DIRECTION ( 'NONE',  ( 1.000000000000000000, 0.000000000000000000, 0.000000000000000000 ) ) ;
#14935=DIRECTION ( 'NONE',  ( 0.000000000000000000, -0.2538061376417695136, -0.9672551082808337197 ) ) ;
#14936=FACE_OUTER_BOUND ( 'NONE', #34201, .T. ) ;
#14962=ORIENTED_EDGE ( 'NONE', *, *, #5723, .F. ) ;
#14974=EDGE_CURVE ( 'NONE', #28609, #30332, #29773, .T. ) ;
#15013=CARTESIAN_POINT ( 'NONE',  ( 70.00000000000001421, 81.48267994499606459, 30.15054357219658954 ) ) ;
#15138=ADVANCED_FACE ( 'NONE', ( #19636 ), #11556, .T. ) ;
#15225=CARTESIAN_POINT ( 'NONE',  ( 70.00001200000001234, -29.17942948312593643, 87.45818687989958562 ) ) ;
#15228=CARTESIAN_POINT ( 'NONE',  ( 63.00000000000001421, -28.31857036507964764, 80.03062855292515110 ) ) ;
#15240=CIRCLE ( 'NONE', #27353, 3.999999999999994671 ) ;
#15305=VECTOR ( 'NONE', #27853, 1000.000000000000114 ) ;
#15381=ORIENTED_EDGE ( 'NONE', *, *, #15388, .F. ) ;
#15388=EDGE_CURVE ( 'NONE', #28924, #28609, #25257, .T. ) ;
#15402=EDGE_CURVE ( 'NONE', #23525, #33336, #32042, .T. ) ;
#15434=PRESENTATION_STYLE_ASSIGNMENT (( #34727 ) ) ;
#15492=ORIENTED_EDGE ( 'NONE', *, *, #17218, .T. ) ;
#15531=ORIENTED_EDGE ( 'NONE', *, *, #22650, .F. ) ;
#15649=DIRECTION ( 'NONE',  ( 0.000000000000000000, 1.000000000000000000, 1.224646799147353207E-16 ) ) ;
#15662=ORIENTED_EDGE ( 'NONE', *, *, #9948, .F. ) ;
#15731=CARTESIAN_POINT ( 'NONE',  ( 70.00000000000001421, 46.66021779527611102, 66.80632251401318911 ) ) ;
#15747=CARTESIAN_POINT ( 'NONE',  ( 70.00000000000001421, 54.25778039068027425, 73.39034659349927381 ) ) ;
#15795=CYLINDRICAL_SURFACE ( 'NONE', #6974, 7.499999999999992895 ) ;
#15855=EDGE_CURVE ( 'NONE', #13276, #23525, #22095, .T. ) ;
#15880=EDGE_CURVE ( 'NONE', #30332, #1954, #22877, .T. ) ;
#15883=CYLINDRICAL_SURFACE ( 'NONE', #13619, 4.000000000000003553 ) ;
#15932=FACE_OUTER_BOUND ( 'NONE', #9827, .T. ) ;
#15965=ORIENTED_EDGE ( 'NONE', *, *, #32177, .T. ) ;
#16022=ORIENTED_EDGE ( 'NONE', *, *, #23090, .F. ) ;
#16033=DIRECTION ( 'NONE',  ( 1.000000000000000000, -0.000000000000000000, -0.000000000000000000 ) ) ;
#16043=CARTESIAN_POINT ( 'NONE',  ( 115.0000000000000000, 81.48267994499606459, 30.15054357219658954 ) ) ;
#16147=ORIENTED_EDGE ( 'NONE', *, *, #32640, .T. ) ;
#16180=DIRECTION ( 'NONE',  ( 0.000000000000000000, -0.2538061376417690140, -0.9672551082808337197 ) ) ;
#16193=CARTESIAN_POINT ( 'NONE',  ( 70.00001200000001234, -21.98076211353320630, 85.52359877559823076 ) ) ;
#16220=EDGE_CURVE ( 'NONE', #9695, #32501, #24068, .T. ) ;
#16247=CARTESIAN_POINT ( 'NONE',  ( 70.00000000000001421, 55.12602127901487847, 78.31438535856030114 ) ) ;
#16281=ORIENTED_EDGE ( 'NONE', *, *, #18394, .F. ) ;
#16303=LINE ( 'NONE', #8387, #10169 ) ;
#16372=ORIENTED_EDGE ( 'NONE', *, *, #3416, .F. ) ;
#16375=AXIS2_PLACEMENT_3D ( 'NONE', #32096, #21090, #24172 ) ;
#16423=CARTESIAN_POINT ( 'NONE',  ( 65.00000000000001421, -31.33892132276156062, 83.40622150580404082 ) ) ;
#16433=UNCERTAINTY_MEASURE_WITH_UNIT (LENGTH_MEASURE( 1.000000000000000082E-05 ), #31754, 'distance_accuracy_value', 'NONE');
#16449=AXIS2_PLACEMENT_3D ( 'NONE', #3683, #6723, #31213 ) ;
#16536=DIRECTION ( 'NONE',  ( 0.000000000000000000, 0.000000000000000000, -1.000000000000000000 ) ) ;
#16551=VERTEX_POINT ( 'NONE', #6553 ) ;
#16588=CARTESIAN_POINT ( 'NONE',  ( 65.00000000000001421, -25.98076211353320986, 77.99999999999992895 ) ) ;
#16617=LINE ( 'NONE', #3489, #6148 ) ;
#16635=CIRCLE ( 'NONE', #24697, 5.000000000000004441 ) ;
#16694=LINE ( 'NONE', #14002, #31623 ) ;
#16703=DIRECTION ( 'NONE',  ( 1.000000000000000000, 0.000000000000000000, 0.000000000000000000 ) ) ;
#16744=DIRECTION ( 'NONE',  ( 0.000000000000000000, 0.000000000000000000, -1.000000000000000000 ) ) ;
#16787=DIRECTION ( 'NONE',  ( -1.000000000000000000, -0.000000000000000000, -0.000000000000000000 ) ) ;
#16814=DIRECTION ( 'NONE',  ( 0.000000000000000000, 0.000000000000000000, -1.000000000000000000 ) ) ;
#16839=DIRECTION ( 'NONE',  ( -1.000000000000000000, -0.000000000000000000, -0.000000000000000000 ) ) ;
#16848=LINE ( 'NONE', #22261, #15305 ) ;
#16849=LINE ( 'NONE', #24977, #13004 ) ;
#16878=DIRECTION ( 'NONE',  ( 0.000000000000000000, 0.000000000000000000, 1.000000000000000000 ) ) ;
#16950=AXIS2_PLACEMENT_3D ( 'NONE', #27676, #24621, #13807 ) ;
#16991=VECTOR ( 'NONE', #17950, 1000.000000000000114 ) ;
#17055=PLANE ( 'NONE',  #5395 ) ;
#17096=LINE ( 'NONE', #30972, #25463 ) ;
#17136=ORIENTED_EDGE ( 'NONE', *, *, #17378, .T. ) ;
#17217=SHAPE_DEFINITION_REPRESENTATION ( #12697, #4547 ) ;
#17218=EDGE_CURVE ( 'NONE', #9695, #9753, #1670, .T. ) ;
#17242=VECTOR ( 'NONE', #33213, 999.9999999999998863 ) ;
#17269=ORIENTED_EDGE ( 'NONE', *, *, #7714, .T. ) ;
#17342=EDGE_LOOP ( 'NONE', ( #1492, #13000 ) ) ;
#17378=EDGE_CURVE ( 'NONE', #33824, #3203, #34486, .T. ) ;
#17459=VECTOR ( 'NONE', #31469, 1000.000000000000114 ) ;
#17479=ORIENTED_EDGE ( 'NONE', *, *, #1843, .F. ) ;
#17524=AXIS2_PLACEMENT_3D ( 'NONE', #10043, #2150, #29669 ) ;
#17634=DIRECTION ( 'NONE',  ( 0.000000000000000000, 0.9672551082808337197, -0.2538061376417689030 ) ) ;
#17641=CARTESIAN_POINT ( 'NONE',  ( 65.00000000000001421, -25.98076211353320986, 84.99999999999994316 ) ) ;
#17642=CARTESIAN_POINT ( 'NONE',  ( 70.00000000000001421, -27.28312344603513040, 77.61394185240837373 ) ) ;
#17690=CARTESIAN_POINT ( 'NONE',  ( 65.00000000000001421, 46.40248769959372055, 64.62118051744215563 ) ) ;
#17723=PLANE ( 'NONE',  #30664 ) ;
#17758=CARTESIAN_POINT ( 'NONE',  ( 70.00001200000001234, -29.47590766695025621, 82.98552407851634882 ) ) ;
#17767=FACE_BOUND ( 'NONE', #12463, .T. ) ;
#17800=LINE ( 'NONE', #20673, #21244 ) ;
#17819=EDGE_CURVE ( 'NONE', #428, #4878, #20630, .T. ) ;
#17931=DIRECTION ( 'NONE',  ( 0.000000000000000000, 0.000000000000000000, 1.000000000000000000 ) ) ;
#17950=DIRECTION ( 'NONE',  ( 0.000000000000000000, 0.9848077530122095746, -0.1736481776669212829 ) ) ;
#17962=DIRECTION ( 'NONE',  ( 0.000000000000000000, 0.000000000000000000, 1.000000000000000000 ) ) ;
#18024=EDGE_CURVE ( 'NONE', #2854, #18471, #24426, .T. ) ;
#18041=ORIENTED_EDGE ( 'NONE', *, *, #26455, .F. ) ;
#18056=DIRECTION ( 'NONE',  ( -1.000000000000000000, -0.000000000000000000, -0.000000000000000000 ) ) ;
#18136=LINE ( 'NONE', #26983, #22134 ) ;
#18186=CYLINDRICAL_SURFACE ( 'NONE', #11318, 5.000000000000004441 ) ;
#18200=CARTESIAN_POINT ( 'NONE',  ( 70.00001200000002655, -24.93377057609608727, 81.10410929332670094 ) ) ;
#18238=FACE_OUTER_BOUND ( 'NONE', #12437, .T. ) ;
#18244=EDGE_CURVE ( 'NONE', #33932, #428, #21084, .T. ) ;
#18292=DIRECTION ( 'NONE',  ( 1.000000000000000000, 0.000000000000000000, 0.000000000000000000 ) ) ;
#18394=EDGE_CURVE ( 'NONE', #19400, #16551, #29576, .T. ) ;
#18446=DIRECTION ( 'NONE',  ( -1.000000000000000000, -0.000000000000000000, -0.000000000000000000 ) ) ;
#18461=CYLINDRICAL_SURFACE ( 'NONE', #261, 7.000000000000006217 ) ;
#18471=VERTEX_POINT ( 'NONE', #2569 ) ;
#18546=CARTESIAN_POINT ( 'NONE',  ( 112.0000000000000000, 81.48267994499606459, 25.65054357219660019 ) ) ;
#18556=CARTESIAN_POINT ( 'NONE',  ( 65.00000000000001421, -35.39471919948800149, 89.19850115919967948 ) ) ;
#18590=CIRCLE ( 'NONE', #7662, 5.000000000000004441 ) ;
#18595=EDGE_CURVE ( 'NONE', #9753, #25616, #5954, .T. ) ;
#18596=VERTEX_POINT ( 'NONE', #3796 ) ;
#18646=EDGE_LOOP ( 'NONE', ( #30992, #20629, #13256, #31970 ) ) ;
#18658=CIRCLE ( 'NONE', #24993, 7.000000000000006217 ) ;
#18670=DIRECTION ( 'NONE',  ( -1.000000000000000000, 0.000000000000000000, 0.000000000000000000 ) ) ;
#18671=LINE ( 'NONE', #2497, #13098 ) ;
#18687=ADVANCED_FACE ( 'NONE', ( #8999 ), #1611, .T. ) ;
#18695=CARTESIAN_POINT ( 'NONE',  ( 65.00000000000001421, -25.98076211353320986, 84.99999999999994316 ) ) ;
#18709=DIRECTION ( 'NONE',  ( 0.000000000000000000, 0.000000000000000000, -1.000000000000000000 ) ) ;
#18838=CARTESIAN_POINT ( 'NONE',  ( 65.00000000000001421, 46.66021779527611102, 66.80632251401318911 ) ) ;
#18907=EDGE_LOOP ( 'NONE', ( #32607, #14733, #27657, #3724, #4373, #18041 ) ) ;
#18928=VECTOR ( 'NONE', #26619, 1000.000000000000000 ) ;
#18985=CARTESIAN_POINT ( 'NONE',  ( 70.00000000000001421, -29.60243954609234507, 93.25429903592612391 ) ) ;
#18997=FACE_OUTER_BOUND ( 'NONE', #23887, .T. ) ;
#19199=CARTESIAN_POINT ( 'NONE',  ( 70.00000600000001327, -25.98076211353320986, 88.99999999999994316 ) ) ;
#19253=CARTESIAN_POINT ( 'NONE',  ( 55.00000000000000711, -25.98076211353320986, 84.99999999999994316 ) ) ;
#19400=VERTEX_POINT ( 'NONE', #22576 ) ;
#19512=LINE ( 'NONE', #22390, #32576 ) ;
#19559=CARTESIAN_POINT ( 'NONE',  ( 55.00000000000000711, -25.98076211353320986, 84.99999999999994316 ) ) ;
#19636=FACE_OUTER_BOUND ( 'NONE', #18646, .T. ) ;
#19666=EDGE_CURVE ( 'NONE', #2565, #28758, #29838, .T. ) ;
#19673=FACE_OUTER_BOUND ( 'NONE', #24669, .T. ) ;
#19751=CARTESIAN_POINT ( 'NONE',  ( 70.00000000000001421, -37.13120097615721704, 79.35042362907756797 ) ) ;
#19757=EDGE_LOOP ( 'NONE', ( #2194, #26333, #4632, #34929 ) ) ;
#19843=DIRECTION ( 'NONE',  ( 0.000000000000000000, 0.000000000000000000, -1.000000000000000000 ) ) ;
#19860=ORIENTED_EDGE ( 'NONE', *, *, #8593, .F. ) ;
#19896=CARTESIAN_POINT ( 'NONE',  ( 112.0000000000000000, 81.48267994499606459, 30.15054357219658954 ) ) ;
#20104=CARTESIAN_POINT ( 'NONE',  ( 65.00000000000001421, 0.000000000000000000, 0.000000000000000000 ) ) ;
#20133=VERTEX_POINT ( 'NONE', #16247 ) ;
#20175=VERTEX_POINT ( 'NONE', #12872 ) ;
#20236=FACE_OUTER_BOUND ( 'NONE', #29775, .T. ) ;
#20406=DIRECTION ( 'NONE',  ( 0.000000000000000000, -0.9848077530122096857, 0.1736481776669211718 ) ) ;
#20504=VECTOR ( 'NONE', #5114, 1000.000000000000000 ) ;
#20543=AXIS2_PLACEMENT_3D ( 'NONE', #982, #11961, #3511 ) ;
#20552=EDGE_LOOP ( 'NONE', ( #6295, #31690, #8577, #5484 ) ) ;
#20613=EDGE_CURVE ( 'NONE', #29380, #28214, #11545, .T. ) ;
#20629=ORIENTED_EDGE ( 'NONE', *, *, #18394, .T. ) ;
#20630=LINE ( 'NONE', #15228, #13090 ) ;
#20654=( NAMED_UNIT ( * ) PLANE_ANGLE_UNIT ( ) SI_UNIT ( $, .RADIAN. ) );
#20673=CARTESIAN_POINT ( 'NONE',  ( 70.00000000000001421, -36.26296008782259861, 84.27446239413865214 ) ) ;
#20694=EDGE_LOOP ( 'NONE', ( #13330, #2593, #7971, #31488, #21146, #15531 ) ) ;
#20788=VERTEX_POINT ( 'NONE', #29305 ) ;
#20802=CARTESIAN_POINT ( 'NONE',  ( 70.00001200000002655, -27.99523803501681130, 81.50485444658289680 ) ) ;
#20817=CARTESIAN_POINT ( 'NONE',  ( 70.00000000000001421, -24.67840078103129997, 92.38605814759151258 ) ) ;
#20840=ORIENTED_EDGE ( 'NONE', *, *, #24868, .T. ) ;
#20930=SURFACE_STYLE_USAGE ( .BOTH. , #26181 ) ;
#20951=CARTESIAN_POINT ( 'NONE',  ( 65.00000000000001421, -24.67840078103129997, 92.38605814759151258 ) ) ;
#21084=LINE ( 'NONE', #34300, #2253 ) ;
#21090=DIRECTION ( 'NONE',  ( 0.000000000000000000, 0.9672551082808338307, -0.2538061376417690695 ) ) ;
#21121=ORIENTED_EDGE ( 'NONE', *, *, #17378, .F. ) ;
#21146=ORIENTED_EDGE ( 'NONE', *, *, #32177, .F. ) ;
#21205=CARTESIAN_POINT ( 'NONE',  ( 55.00000000000000711, -27.93100416606587899, 81.50764321173589622 ) ) ;
#21221=DIRECTION ( 'NONE',  ( 0.000000000000000000, 0.000000000000000000, 1.000000000000000000 ) ) ;
#21244=VECTOR ( 'NONE', #1255, 1000.000000000000000 ) ;
#21255=CARTESIAN_POINT ( 'NONE',  ( 70.00001200000001234, -22.48561656011616350, 87.01447592148353749 ) ) ;
#21307=AXIS2_PLACEMENT_3D ( 'NONE', #26589, #12725, #18292 ) ;
#21358=ADVANCED_FACE ( 'NONE', ( #1182 ), #17723, .T. ) ;
#21410=CARTESIAN_POINT ( 'NONE',  ( 55.00000000000000711, -25.98076211353320986, 84.99999999999994316 ) ) ;
#21463=EDGE_LOOP ( 'NONE', ( #25990, #28789, #28463, #33102 ) ) ;
#21475=CARTESIAN_POINT ( 'NONE',  ( 55.00000000000000711, -25.98076211353320986, 84.99999999999994316 ) ) ;
#21555=CARTESIAN_POINT ( 'NONE',  ( 115.0000000000000000, 81.48267994499606459, 30.15054357219658954 ) ) ;
#21588=EDGE_LOOP ( 'NONE', ( #33355, #7484, #10383, #10469 ) ) ;
#21659=AXIS2_PLACEMENT_3D ( 'NONE', #156, #24479, #16878 ) ;
#21702=ORIENTED_EDGE ( 'NONE', *, *, #13307, .F. ) ;
#21774=VERTEX_POINT ( 'NONE', #6707 ) ;
#21823=EDGE_CURVE ( 'NONE', #30224, #14334, #28688, .T. ) ;
#21862=ORIENTED_EDGE ( 'NONE', *, *, #15402, .F. ) ;
#21910=CARTESIAN_POINT ( 'NONE',  ( 55.00000000000000711, -25.98076211353320986, 77.99999999999992895 ) ) ;
#22062=AXIS2_PLACEMENT_3D ( 'NONE', #636, #20406, #1354 ) ;
#22090=CARTESIAN_POINT ( 'NONE',  ( 65.00000000000001421, -27.93100416606583636, 81.50764321173598148 ) ) ;
#22095=LINE ( 'NONE', #25171, #26344 ) ;
#22100=ORIENTED_EDGE ( 'NONE', *, *, #23726, .T. ) ;
#22118=FACE_OUTER_BOUND ( 'NONE', #20694, .T. ) ;
#22134=VECTOR ( 'NONE', #18670, 1000.000000000000000 ) ;
#22261=CARTESIAN_POINT ( 'NONE',  ( 65.00000000000001421, -28.31857036507964764, 80.03062855292515110 ) ) ;
#22284=ADVANCED_FACE ( 'NONE', ( #14573 ), #23411, .T. ) ;
#22299=LINE ( 'NONE', #19751, #8939 ) ;
#22363=PRODUCT_DEFINITION_CONTEXT ( 'detailed design', #8498, 'design' ) ;
#22390=CARTESIAN_POINT ( 'NONE',  ( 65.00000000000001421, -37.13120097615721704, 79.35042362907756797 ) ) ;
#22446=ORIENTED_EDGE ( 'NONE', *, *, #2954, .F. ) ;
#22527=ADVANCED_FACE ( 'NONE', ( #20236 ), #14486, .T. ) ;
#22555=ORIENTED_EDGE ( 'NONE', *, *, #31805, .T. ) ;
#22576=CARTESIAN_POINT ( 'NONE',  ( 65.00000000000001421, 58.35354061212520804, 76.25822877525452270 ) ) ;
#22650=EDGE_CURVE ( 'NONE', #18596, #34599, #32136, .T. ) ;
#22682=PRODUCT_DEFINITION ( 'UNKNOWN', '', #25884, #22363 ) ;
#22698=CIRCLE ( 'NONE', #24448, 5.000000000000004441 ) ;
#22699=VERTEX_POINT ( 'NONE', #2809 ) ;
#22727=CIRCLE ( 'NONE', #5509, 7.000000000000006217 ) ;
#22858=DIRECTION ( 'NONE',  ( 0.000000000000000000, 0.000000000000000000, 1.000000000000000000 ) ) ;
#22877=CIRCLE ( 'NONE', #30358, 4.000000000000003553 ) ;
#22923=PLANE ( 'NONE',  #16449 ) ;
#22934=( LENGTH_UNIT ( ) NAMED_UNIT ( * ) SI_UNIT ( .MILLI., .METRE. ) );
#23057=( GEOMETRIC_REPRESENTATION_CONTEXT ( 3 ) GLOBAL_UNCERTAINTY_ASSIGNED_CONTEXT ( ( #33022 ) ) GLOBAL_UNIT_ASSIGNED_CONTEXT ( ( #22934, #14299, #11601 ) ) REPRESENTATION_CONTEXT ( 'NONE', 'WORKASPACE' ) );
#23085=DIRECTION ( 'NONE',  ( -1.000000000000000000, -0.000000000000000000, -0.000000000000000000 ) ) ;
#23090=EDGE_CURVE ( 'NONE', #16551, #20133, #31788, .T. ) ;
#23121=VECTOR ( 'NONE', #18446, 1000.000000000000000 ) ;
#23141=CARTESIAN_POINT ( 'NONE',  ( 70.00000000000001421, 46.66021779527611102, 66.80632251401318911 ) ) ;
#23169=CARTESIAN_POINT ( 'NONE',  ( 70.00001200000001234, -28.43894899343287364, 88.19866736959266973 ) ) ;
#23220=CARTESIAN_POINT ( 'NONE',  ( 55.00000000000000711, -28.31857036507964764, 80.03062855292515110 ) ) ;
#23254=ORIENTED_EDGE ( 'NONE', *, *, #27033, .F. ) ;
#23311=PLANE ( 'NONE',  #32487 ) ;
#23318=DIRECTION ( 'NONE',  ( 0.000000000000000000, 0.5735764363510502672, -0.8191520442889889120 ) ) ;
#23325=ORIENTED_EDGE ( 'NONE', *, *, #143, .F. ) ;
#23343=CARTESIAN_POINT ( 'NONE',  ( 70.00001200000001234, -27.99523803501680419, 88.49514555341693267 ) ) ;
#23356=PLANE ( 'NONE',  #8231 ) ;
#23411=PLANE ( 'NONE',  #13059 ) ;
#23443=EDGE_LOOP ( 'NONE', ( #25350, #13044, #1496, #23325 ) ) ;
#23525=VERTEX_POINT ( 'NONE', #5388 ) ;
#23554=CARTESIAN_POINT ( 'NONE',  ( 115.0000000000000000, 81.48267994499606459, 25.65054357219660019 ) ) ;
#23637=FACE_OUTER_BOUND ( 'NONE', #34008, .T. ) ;
#23655=CARTESIAN_POINT ( 'NONE',  ( 70.00000000000001421, 81.48267994499606459, 37.65054357219658243 ) ) ;
#23657=LINE ( 'NONE', #13034, #33544 ) ;
#23669=DIRECTION ( 'NONE',  ( 1.000000000000000000, 0.000000000000000000, 0.000000000000000000 ) ) ;
#23726=EDGE_CURVE ( 'NONE', #19400, #22699, #31277, .T. ) ;
#23737=SURFACE_STYLE_FILL_AREA ( #346 ) ;
#23797=CARTESIAN_POINT ( 'NONE',  ( 70.00001200000001234, -22.08487140685993921, 83.95300846256282057 ) ) ;
#23821=CARTESIAN_POINT ( 'NONE',  ( 65.00000000000001421, -32.20716221109618260, 78.48218274074299927 ) ) ;
#23832=DIRECTION ( 'NONE',  ( 0.000000000000000000, 0.000000000000000000, 1.000000000000000000 ) ) ;
#23887=EDGE_LOOP ( 'NONE', ( #16022, #16281, #23254, #1271 ) ) ;
#23921=SURFACE_SIDE_STYLE ('',( #23737 ) ) ;
#23961=ORIENTED_EDGE ( 'NONE', *, *, #26503, .F. ) ;
#23964=CARTESIAN_POINT ( 'NONE',  ( 55.00000000000000711, -25.01350700525240356, 84.74619386235809770 ) ) ;
#24002=EDGE_CURVE ( 'NONE', #1954, #4878, #10033, .T. ) ;
#24068=CIRCLE ( 'NONE', #14838, 5.000000000000004441 ) ;
#24153=CARTESIAN_POINT ( 'NONE',  ( 70.00001200000001234, -23.52257523363354608, 88.19866736959268394 ) ) ;
#24172=DIRECTION ( 'NONE',  ( 0.000000000000000000, 0.2538061376417690140, 0.9672551082808337197 ) ) ;
#24235=DIRECTION ( 'NONE',  ( 0.000000000000000000, 0.000000000000000000, 1.000000000000000000 ) ) ;
#24276=FACE_OUTER_BOUND ( 'NONE', #20552, .T. ) ;
#24297=DIRECTION ( 'NONE',  ( 0.000000000000000000, 0.000000000000000000, 1.000000000000000000 ) ) ;
#24333=CARTESIAN_POINT ( 'NONE',  ( 70.00001200000001234, -22.78209474394047973, 82.54181312010027227 ) ) ;
#24344=CARTESIAN_POINT ( 'NONE',  ( 70.00000000000001421, 58.35354061212520804, 76.25822877525452270 ) ) ;
#24425=ADVANCED_FACE ( 'NONE', ( #23637 ), #2232, .F. ) ;
#24426=LINE ( 'NONE', #18838, #3910 ) ;
#24448=AXIS2_PLACEMENT_3D ( 'NONE', #5272, #33331, #24528 ) ;
#24479=DIRECTION ( 'NONE',  ( -1.000000000000000000, 0.000000000000000000, 0.000000000000000000 ) ) ;
#24506=CARTESIAN_POINT ( 'NONE',  ( 70.00001200000001234, -22.48561656011616705, 82.98552407851633461 ) ) ;
#24528=DIRECTION ( 'NONE',  ( 0.000000000000000000, 0.000000000000000000, 1.000000000000000000 ) ) ;
#24533=AXIS2_PLACEMENT_3D ( 'NONE', #24831, #27882, #515 ) ;
#24579=DIRECTION ( 'NONE',  ( -1.000000000000000000, 0.000000000000000000, 0.000000000000000000 ) ) ;
#24595=CARTESIAN_POINT ( 'NONE',  ( 112.0000000000000000, 81.48267994499606459, 34.65054357219658243 ) ) ;
#24621=DIRECTION ( 'NONE',  ( -1.000000000000000000, 0.000000000000000000, 0.000000000000000000 ) ) ;
#24635=EDGE_CURVE ( 'NONE', #35307, #29380, #22698, .T. ) ;
#24638=DIRECTION ( 'NONE',  ( 0.000000000000000000, 0.000000000000000000, -1.000000000000000000 ) ) ;
#24663=DIRECTION ( 'NONE',  ( 0.000000000000000000, 0.1736481776669211718, 0.9848077530122096857 ) ) ;
#24669=EDGE_LOOP ( 'NONE', ( #27204, #17136 ) ) ;
#24697=AXIS2_PLACEMENT_3D ( 'NONE', #32276, #5445, #2403 ) ;
#24790=DIRECTION ( 'NONE',  ( 0.000000000000000000, 4.163336342344333082E-15, 1.000000000000000000 ) ) ;
#24831=CARTESIAN_POINT ( 'NONE',  ( 65.00000000000001421, 81.48267994499606459, 30.15054357219658954 ) ) ;
#24868=EDGE_CURVE ( 'NONE', #13276, #33932, #15240, .T. ) ;
#24977=CARTESIAN_POINT ( 'NONE',  ( 65.00000000000001421, 49.63000703270403591, 62.56502393413636298 ) ) ;
#24993=AXIS2_PLACEMENT_3D ( 'NONE', #1235, #14894, #33823 ) ;
#25002=DIRECTION ( 'NONE',  ( 0.000000000000000000, -0.2538061376417689030, -0.9672551082808337197 ) ) ;
#25007=B_SPLINE_CURVE_WITH_KNOTS ( 'NONE', 3,
 ( #12553, #33988, #6962, #23343, #23169, #15225, #31458, #26234, #34343, #31627, #1573, #17758, #3932, #9839, #20802, #25891, #28582, #9670 ),
 .UNSPECIFIED., .F., .F.,
 ( 4, 2, 2, 2, 2, 2, 2, 2, 4 ),
 ( 0.5000000000000000000, 0.5625000000000000000, 0.6250000000000000000, 0.6875000000000000000, 0.7500000000000000000, 0.8125000000000000000, 0.8750000000000000000, 0.9375000000000000000, 1.000000000000000000 ),
 .UNSPECIFIED. ) ;
#25010=DIRECTION ( 'NONE',  ( 0.000000000000000000, 0.000000000000000000, 1.000000000000000000 ) ) ;
#25065=EDGE_CURVE ( 'NONE', #14334, #7205, #22727, .T. ) ;
#25139=UNCERTAINTY_MEASURE_WITH_UNIT (LENGTH_MEASURE( 1.000000000000000082E-05 ), #7166, 'distance_accuracy_value', 'NONE');
#25148=AXIS2_PLACEMENT_3D ( 'NONE', #32708, #27139, #13280 ) ;
#25171=CARTESIAN_POINT ( 'NONE',  ( 75.00000000000002842, -25.99649394950422021, 81.00003093645240426 ) ) ;
#25257=B_SPLINE_CURVE_WITH_KNOTS ( 'NONE', 3,
 ( #32251, #13180, #18200, #13523, #29910, #24333, #24506, #23797, #29211, #16193, #34779, #21255, #5078, #24153, #32428, #2380, #7576, #4730 ),
 .UNSPECIFIED., .F., .F.,
 ( 4, 2, 2, 2, 2, 2, 2, 2, 4 ),
 ( 0.000000000000000000, 0.06250000000000000000, 0.1250000000000000000, 0.1875000000000000000, 0.2500000000000000000, 0.3125000000000000000, 0.3750000000000000000, 0.4375000000000000000, 0.5000000000000000000 ),
 .UNSPECIFIED. ) ;
#25278=ORIENTED_EDGE ( 'NONE', *, *, #29434, .F. ) ;
#25293=CYLINDRICAL_SURFACE ( 'NONE', #20543, 7.000000000000006217 ) ;
#25350=ORIENTED_EDGE ( 'NONE', *, *, #3993, .F. ) ;
#25400=DIRECTION ( 'NONE',  ( -0.000000000000000000, 0.1736481776669212829, 0.9848077530122096857 ) ) ;
#25404=CARTESIAN_POINT ( 'NONE',  ( 70.00000000000001421, 46.40248769959371344, 64.62118051744215563 ) ) ;
#25406=DIRECTION ( 'NONE',  ( 1.000000000000000000, 0.000000000000000000, 0.000000000000000000 ) ) ;
#25441=EDGE_CURVE ( 'NONE', #13682, #20133, #1767, .T. ) ;
#25456=LINE ( 'NONE', #776, #26910 ) ;
#25461=DIRECTION ( 'NONE',  ( 1.000000000000000000, 0.000000000000000000, 0.000000000000000000 ) ) ;
#25463=VECTOR ( 'NONE', #3269, 1000.000000000000114 ) ;
#25476=FILL_AREA_STYLE_COLOUR ( '', #6385 ) ;
#25478=ORIENTED_EDGE ( 'NONE', *, *, #10829, .F. ) ;
#25512=AXIS2_PLACEMENT_3D ( 'NONE', #14357, #10970, #27879 ) ;
#25528=CARTESIAN_POINT ( 'NONE',  ( 65.00000000000001421, 58.94749845961094792, 75.40996905927893579 ) ) ;
#25576=DIRECTION ( 'NONE',  ( 0.000000000000000000, -0.9848077530122095746, 0.1736481776669212551 ) ) ;
#25616=VERTEX_POINT ( 'NONE', #27675 ) ;
#25653=ORIENTED_EDGE ( 'NONE', *, *, #26455, .T. ) ;
#25660=ORIENTED_EDGE ( 'NONE', *, *, #8641, .T. ) ;
#25679=DIRECTION ( 'NONE',  ( -1.000000000000000000, 0.000000000000000000, 0.000000000000000000 ) ) ;
#25699=ORIENTED_EDGE ( 'NONE', *, *, #18595, .T. ) ;
#25715=AXIS2_PLACEMENT_3D ( 'NONE', #13797, #16703, #16536 ) ;
#25884=PRODUCT_DEFINITION_FORMATION_WITH_SPECIFIED_SOURCE ( 'ANY', '', #31654, .NOT_KNOWN. ) ;
#25891=CARTESIAN_POINT ( 'NONE',  ( 70.00001200000004076, -27.02775365097033244, 81.10410929332667251 ) ) ;
#25901=FACE_OUTER_BOUND ( 'NONE', #31344, .T. ) ;
#25950=VERTEX_POINT ( 'NONE', #9284 ) ;
#25988=DIRECTION ( 'NONE',  ( 1.000000000000000000, -0.000000000000000000, -0.000000000000000000 ) ) ;
#25990=ORIENTED_EDGE ( 'NONE', *, *, #25441, .T. ) ;
#26100=VERTEX_POINT ( 'NONE', #10180 ) ;
#26148=DIRECTION ( 'NONE',  ( 0.000000000000000000, 0.9848077530122092416, -0.1736481776669233923 ) ) ;
#26181=SURFACE_SIDE_STYLE ('',( #1165 ) ) ;
#26234=CARTESIAN_POINT ( 'NONE',  ( 70.00001200000001234, -29.87665282020647695, 86.04699153743705153 ) ) ;
#26286=EDGE_CURVE ( 'NONE', #34443, #29380, #11238, .T. ) ;
#26333=ORIENTED_EDGE ( 'NONE', *, *, #17819, .F. ) ;
#26344=VECTOR ( 'NONE', #8236, 1000.000000000000000 ) ;
#26349=COLOUR_RGB ( '', 0.08235294, 0.09019608, 0.10196078) ;
#26455=EDGE_CURVE ( 'NONE', #23525, #28758, #32413, .T. ) ;
#26484=VERTEX_POINT ( 'NONE', #7563 ) ;
#26503=EDGE_CURVE ( 'NONE', #33824, #21774, #8219, .T. ) ;
#26509=DIRECTION ( 'NONE',  ( 1.000000000000000000, 0.000000000000000000, 0.000000000000000000 ) ) ;
#26589=CARTESIAN_POINT ( 'NONE',  ( 0.000000000000000000, 0.000000000000000000, 0.000000000000000000 ) ) ;
#26619=DIRECTION ( 'NONE',  ( -1.000000000000000000, 0.000000000000000000, 0.000000000000000000 ) ) ;
#26620=ORIENTED_EDGE ( 'NONE', *, *, #5723, .T. ) ;
#26712=ORIENTED_EDGE ( 'NONE', *, *, #20613, .T. ) ;
#26910=VECTOR ( 'NONE', #6530, 1000.000000000000000 ) ;
#26959=EDGE_CURVE ( 'NONE', #20133, #20788, #18136, .T. ) ;
#26969=VECTOR ( 'NONE', #16033, 1000.000000000000000 ) ;
#26983=CARTESIAN_POINT ( 'NONE',  ( 70.00000000000001421, 55.12602127901489268, 78.31438535856030114 ) ) ;
#26990=ORIENTED_EDGE ( 'NONE', *, *, #9939, .T. ) ;
#27033=EDGE_CURVE ( 'NONE', #20788, #19400, #3746, .T. ) ;
#27137=DIRECTION ( 'NONE',  ( -1.000000000000000000, 0.000000000000000000, -0.000000000000000000 ) ) ;
#27139=DIRECTION ( 'NONE',  ( 1.000000000000000000, 0.000000000000000000, 0.000000000000000000 ) ) ;
#27168=DIRECTION ( 'NONE',  ( 1.000000000000000000, 0.000000000000000000, 0.000000000000000000 ) ) ;
#27204=ORIENTED_EDGE ( 'NONE', *, *, #904, .T. ) ;
#27215=DIRECTION ( 'NONE',  ( 0.000000000000000000, 0.000000000000000000, -1.000000000000000000 ) ) ;
#27260=DIRECTION ( 'NONE',  ( -1.000000000000000000, 0.000000000000000000, 0.000000000000000000 ) ) ;
#27312=AXIS2_PLACEMENT_3D ( 'NONE', #27549, #30423, #25010 ) ;
#27328=DIRECTION ( 'NONE',  ( 1.000000000000000000, -0.000000000000000000, -0.000000000000000000 ) ) ;
#27353=AXIS2_PLACEMENT_3D ( 'NONE', #17641, #28644, #14935 ) ;
#27372=VECTOR ( 'NONE', #23085, 1000.000000000000000 ) ;
#27385=LINE ( 'NONE', #11683, #35523 ) ;
#27465=CARTESIAN_POINT ( 'NONE',  ( 65.00000000000001421, -28.31857036507964764, 80.03062855292515110 ) ) ;
#27549=CARTESIAN_POINT ( 'NONE',  ( 115.0000000000000000, 81.48267994499606459, 30.15054357219658954 ) ) ;
#27657=ORIENTED_EDGE ( 'NONE', *, *, #15880, .T. ) ;
#27675=CARTESIAN_POINT ( 'NONE',  ( 70.00000000000001421, 46.40248769959372055, 64.62118051744215563 ) ) ;
#27676=CARTESIAN_POINT ( 'NONE',  ( 70.00000000000001421, 81.48267994499606459, 30.15054357219658954 ) ) ;
#27751=AXIS2_PLACEMENT_3D ( 'NONE', #5787, #25406, #16744 ) ;
#27825=EDGE_LOOP ( 'NONE', ( #11081, #5849, #4565, #14056 ) ) ;
#27853=DIRECTION ( 'NONE',  ( 0.000000000000000000, 0.9672551082808337197, -0.2538061376417689030 ) ) ;
#27860=ORIENTED_EDGE ( 'NONE', *, *, #7714, .F. ) ;
#27879=DIRECTION ( 'NONE',  ( 0.000000000000000000, 0.000000000000000000, 1.000000000000000000 ) ) ;
#27882=DIRECTION ( 'NONE',  ( -1.000000000000000000, 0.000000000000000000, 0.000000000000000000 ) ) ;
#27885=LINE ( 'NONE', #3229, #33064 ) ;
#27993=CARTESIAN_POINT ( 'NONE',  ( 65.00000000000001421, -26.38406014851796400, 79.52301627764160230 ) ) ;
#28034=CARTESIAN_POINT ( 'NONE',  ( 70.00000000000001421, -32.20716221109618260, 78.48218274074299927 ) ) ;
#28035=EDGE_CURVE ( 'NONE', #20175, #26484, #22299, .T. ) ;
#28124=CARTESIAN_POINT ( 'NONE',  ( 70.00000000000001421, 58.94749845961094792, 75.40996905927893579 ) ) ;
#28197=DIRECTION ( 'NONE',  ( -1.000000000000000000, 0.000000000000000000, 0.000000000000000000 ) ) ;
#28214=VERTEX_POINT ( 'NONE', #12032 ) ;
#28238=( GEOMETRIC_REPRESENTATION_CONTEXT ( 3 ) GLOBAL_UNCERTAINTY_ASSIGNED_CONTEXT ( ( #16433 ) ) GLOBAL_UNIT_ASSIGNED_CONTEXT ( ( #31754, #1888, #9617 ) ) REPRESENTATION_CONTEXT ( 'NONE', 'WORKASPACE' ) );
#28314=CIRCLE ( 'NONE', #12768, 7.499999999999992895 ) ;
#28343=EDGE_LOOP ( 'NONE', ( #6022, #16147, #29827, #13666 ) ) ;
#28347=AXIS2_PLACEMENT_3D ( 'NONE', #31380, #25988, #1314 ) ;
#28463=ORIENTED_EDGE ( 'NONE', *, *, #9282, .F. ) ;
#28526=EDGE_LOOP ( 'NONE', ( #21702, #22555, #11133, #14962, #14871, #19860 ) ) ;
#28582=CARTESIAN_POINT ( 'NONE',  ( 70.00001200000001234, -26.50436088913151522, 80.99999999999990052 ) ) ;
#28593=DIRECTION ( 'NONE',  ( 0.000000000000000000, 0.000000000000000000, 1.000000000000000000 ) ) ;
#28609=VERTEX_POINT ( 'NONE', #19199 ) ;
#28644=DIRECTION ( 'NONE',  ( -1.000000000000000000, 0.000000000000000000, 0.000000000000000000 ) ) ;
#28668=EDGE_LOOP ( 'NONE', ( #17479, #13521, #5971, #6145 ) ) ;
#28688=LINE ( 'NONE', #31905, #27372 ) ;
#28695=FACE_OUTER_BOUND ( 'NONE', #28668, .T. ) ;
#28758=VERTEX_POINT ( 'NONE', #31605 ) ;
#28769=DIRECTION ( 'NONE',  ( 0.000000000000000000, 0.000000000000000000, 1.000000000000000000 ) ) ;
#28789=ORIENTED_EDGE ( 'NONE', *, *, #26959, .T. ) ;
#28867=CYLINDRICAL_SURFACE ( 'NONE', #3232, 4.999999999999997335 ) ;
#28924=VERTEX_POINT ( 'NONE', #32144 ) ;
#29188=DIRECTION ( 'NONE',  ( -0.000000000000000000, 0.1736481776669234200, 0.9848077530122093526 ) ) ;
#29197=DIRECTION ( 'NONE',  ( -1.000000000000000000, 0.000000000000000000, 0.000000000000000000 ) ) ;
#29211=CARTESIAN_POINT ( 'NONE',  ( 70.00001200000001234, -21.98076211353320630, 84.47640122440162713 ) ) ;
#29277=ORIENTED_EDGE ( 'NONE', *, *, #143, .T. ) ;
#29294=DIRECTION ( 'NONE',  ( -1.000000000000000000, 0.000000000000000000, 0.000000000000000000 ) ) ;
#29305=CARTESIAN_POINT ( 'NONE',  ( 65.00000000000001421, 55.12602127901487847, 78.31438535856030114 ) ) ;
#29380=VERTEX_POINT ( 'NONE', #5075 ) ;
#29434=EDGE_CURVE ( 'NONE', #26484, #35307, #27385, .T. ) ;
#29471=ADVANCED_FACE ( 'NONE', ( #11166, #33475 ), #32955, .F. ) ;
#29576=LINE ( 'NONE', #24344, #26969 ) ;
#29648=DIRECTION ( 'NONE',  ( 0.000000000000000000, 0.000000000000000000, 1.000000000000000000 ) ) ;
#29669=DIRECTION ( 'NONE',  ( 0.000000000000000000, 0.000000000000000000, 1.000000000000000000 ) ) ;
#29729=CIRCLE ( 'NONE', #25715, 7.000000000000006217 ) ;
#29773=LINE ( 'NONE', #2413, #20504 ) ;
#29775=EDGE_LOOP ( 'NONE', ( #2745, #130, #13750, #25278 ) ) ;
#29808=CARTESIAN_POINT ( 'NONE',  ( 112.0000000000000000, 81.48267994499606459, 30.15054357219658954 ) ) ;
#29823=DIRECTION ( 'NONE',  ( -1.000000000000000000, 0.000000000000000000, 0.000000000000000000 ) ) ;
#29827=ORIENTED_EDGE ( 'NONE', *, *, #28035, .T. ) ;
#29838=LINE ( 'NONE', #32515, #8024 ) ;
#29910=CARTESIAN_POINT ( 'NONE',  ( 70.00001200000001234, -23.52257523363354252, 81.80133263040720237 ) ) ;
#29934=DIRECTION ( 'NONE',  ( 0.000000000000000000, 0.9848077530122092416, -0.1736481776669233923 ) ) ;
#29964=CARTESIAN_POINT ( 'NONE',  ( 65.00000000000001421, -36.26296008782259861, 84.27446239413865214 ) ) ;
#30051=FACE_OUTER_BOUND ( 'NONE', #1269, .T. ) ;
#30094=ORIENTED_EDGE ( 'NONE', *, *, #2663, .F. ) ;
#30103=VECTOR ( 'NONE', #11826, 999.9999999999998863 ) ;
#30106=LINE ( 'NONE', #13728, #14339 ) ;
#30224=VERTEX_POINT ( 'NONE', #33799 ) ;
#30332=VERTEX_POINT ( 'NONE', #56 ) ;
#30358=AXIS2_PLACEMENT_3D ( 'NONE', #19559, #27168, #24638 ) ;
#30388=ORIENTED_EDGE ( 'NONE', *, *, #3993, .T. ) ;
#30423=DIRECTION ( 'NONE',  ( -1.000000000000000000, -0.000000000000000000, -0.000000000000000000 ) ) ;
#30645=DIRECTION ( 'NONE',  ( -0.000000000000000000, 0.8191520442889889120, 0.5735764363510502672 ) ) ;
#30664=AXIS2_PLACEMENT_3D ( 'NONE', #7102, #6927, #7282 ) ;
#30666=AXIS2_PLACEMENT_3D ( 'NONE', #30892, #28197, #3368 ) ;
#30675=AXIS2_PLACEMENT_3D ( 'NONE', #16043, #32279, #13021 ) ;
#30687=PLANE ( 'NONE',  #13824 ) ;
#30696=FACE_OUTER_BOUND ( 'NONE', #12858, .T. ) ;
#30728=DIRECTION ( 'NONE',  ( -1.000000000000000000, 0.000000000000000000, 0.000000000000000000 ) ) ;
#30776=DIRECTION ( 'NONE',  ( 1.000000000000000000, 0.000000000000000000, 0.000000000000000000 ) ) ;
#30872=CIRCLE ( 'NONE', #21659, 7.499999999999992895 ) ;
#30892=CARTESIAN_POINT ( 'NONE',  ( 70.00000000000001421, -30.47068043442695284, 88.33026027086506815 ) ) ;
#30925=ORIENTED_EDGE ( 'NONE', *, *, #14553, .T. ) ;
#30970=CARTESIAN_POINT ( 'NONE',  ( 112.0000000000000000, 81.48267994499606459, 30.15054357219658954 ) ) ;
#30972=CARTESIAN_POINT ( 'NONE',  ( 65.00000000000001421, -26.38406014851796400, 79.52301627764160230 ) ) ;
#30992=ORIENTED_EDGE ( 'NONE', *, *, #23726, .F. ) ;
#31108=DIRECTION ( 'NONE',  ( 0.000000000000000000, 0.000000000000000000, 1.000000000000000000 ) ) ;
#31187=AXIS2_PLACEMENT_3D ( 'NONE', #21475, #23669, #10158 ) ;
#31213=DIRECTION ( 'NONE',  ( 0.000000000000000000, 0.000000000000000000, 1.000000000000000000 ) ) ;
#31277=LINE ( 'NONE', #25528, #30103 ) ;
#31290=ADVANCED_FACE ( 'NONE', ( #35106 ), #15795, .T. ) ;
#31344=EDGE_LOOP ( 'NONE', ( #22100, #34962, #4235, #5424, #35280, #4503, #3388, #30925, #10856, #26712, #3276, #35287 ) ) ;
#31380=CARTESIAN_POINT ( 'NONE',  ( 70.00000000000001421, 54.25778039068027425, 73.39034659349927381 ) ) ;
#31386=DIRECTION ( 'NONE',  ( -1.000000000000000000, 0.000000000000000000, 0.000000000000000000 ) ) ;
#31389=FACE_OUTER_BOUND ( 'NONE', #10625, .T. ) ;
#31458=CARTESIAN_POINT ( 'NONE',  ( 70.00001200000001234, -29.47590766695025266, 87.01447592148352328 ) ) ;
#31469=DIRECTION ( 'NONE',  ( 0.000000000000000000, -0.2538061376417690140, -0.9672551082808337197 ) ) ;
#31488=ORIENTED_EDGE ( 'NONE', *, *, #9541, .F. ) ;
#31592=AXIS2_PLACEMENT_3D ( 'NONE', #8070, #5038, #24297 ) ;
#31605=CARTESIAN_POINT ( 'NONE',  ( 55.00000000000000711, -26.38406014851796400, 79.52301627764160230 ) ) ;
#31623=VECTOR ( 'NONE', #14179, 1000.000000000000000 ) ;
#31627=CARTESIAN_POINT ( 'NONE',  ( 70.00001200000001234, -29.98076211353320986, 84.47640122440162713 ) ) ;
#31654=PRODUCT ( 'handle', 'handle', '', ( #9308 ) ) ;
#31670=ORIENTED_EDGE ( 'NONE', *, *, #9948, .T. ) ;
#31678=LINE ( 'NONE', #23220, #9955 ) ;
#31685=CARTESIAN_POINT ( 'NONE',  ( 55.00000000000000711, -28.31857036507964764, 80.03062855292515110 ) ) ;
#31690=ORIENTED_EDGE ( 'NONE', *, *, #9939, .F. ) ;
#31754=( LENGTH_UNIT ( ) NAMED_UNIT ( * ) SI_UNIT ( .MILLI., .METRE. ) );
#31788=CIRCLE ( 'NONE', #28347, 5.000000000000004441 ) ;
#31805=EDGE_CURVE ( 'NONE', #21774, #18596, #32298, .T. ) ;
#31822=CIRCLE ( 'NONE', #14559, 5.000000000000004441 ) ;
#31872=DIRECTION ( 'NONE',  ( 0.000000000000000000, 0.000000000000000000, 1.000000000000000000 ) ) ;
#31905=CARTESIAN_POINT ( 'NONE',  ( 65.00000000000001421, -25.98076211353320986, 91.99999999999994316 ) ) ;
#31929=FILL_AREA_STYLE ('',( #25476 ) ) ;
#31970=ORIENTED_EDGE ( 'NONE', *, *, #9541, .T. ) ;
#32042=CIRCLE ( 'NONE', #11357, 4.000000000000003553 ) ;
#32096=CARTESIAN_POINT ( 'NONE',  ( 63.00000000000001421, -25.01350700525240356, 84.74619386235809770 ) ) ;
#32136=LINE ( 'NONE', #7466, #23121 ) ;
#32144=CARTESIAN_POINT ( 'NONE',  ( 70.00000600000001327, -25.98076211353320986, 80.99999999999992895 ) ) ;
#32177=EDGE_CURVE ( 'NONE', #34599, #5076, #28314, .T. ) ;
#32251=CARTESIAN_POINT ( 'NONE',  ( 70.00000600000001327, -25.98076211353320986, 80.99999999999992895 ) ) ;
#32276=CARTESIAN_POINT ( 'NONE',  ( 70.00000000000001421, -30.47068043442695284, 88.33026027086506815 ) ) ;
#32279=DIRECTION ( 'NONE',  ( 1.000000000000000000, -0.000000000000000000, -0.000000000000000000 ) ) ;
#32298=CIRCLE ( 'NONE', #6409, 7.499999999999992895 ) ;
#32390=EDGE_CURVE ( 'NONE', #7205, #14334, #8758, .T. ) ;
#32413=LINE ( 'NONE', #23964, #7063 ) ;
#32414=ORIENTED_EDGE ( 'NONE', *, *, #7310, .F. ) ;
#32428=CARTESIAN_POINT ( 'NONE',  ( 70.00001200000002655, -23.96628619204960486, 88.49514555341697530 ) ) ;
#32446=AXIS2_PLACEMENT_3D ( 'NONE', #17642, #29188, #12616 ) ;
#32487=AXIS2_PLACEMENT_3D ( 'NONE', #15731, #4617, #34312 ) ;
#32497=ADVANCED_FACE ( 'NONE', ( #14562 ), #5473, .T. ) ;
#32501=VERTEX_POINT ( 'NONE', #29964 ) ;
#32511=ORIENTED_EDGE ( 'NONE', *, *, #23090, .T. ) ;
#32515=CARTESIAN_POINT ( 'NONE',  ( 63.00000000000001421, -26.38406014851796400, 79.52301627764160230 ) ) ;
#32519=CYLINDRICAL_SURFACE ( 'NONE', #25148, 5.000000000000004441 ) ;
#32555=ORIENTED_EDGE ( 'NONE', *, *, #19666, .F. ) ;
#32576=VECTOR ( 'NONE', #13948, 1000.000000000000000 ) ;
#32578=CARTESIAN_POINT ( 'NONE',  ( 70.00000000000001421, 87.62632027716348659, 34.45236684482946288 ) ) ;
#32607=ORIENTED_EDGE ( 'NONE', *, *, #15402, .T. ) ;
#32640=EDGE_CURVE ( 'NONE', #32501, #20175, #17800, .T. ) ;
#32708=CARTESIAN_POINT ( 'NONE',  ( 70.00000000000001421, -31.33892132276156062, 83.40622150580404082 ) ) ;
#32855=ORIENTED_EDGE ( 'NONE', *, *, #15388, .T. ) ;
#32877=ADVANCED_FACE ( 'NONE', ( #30051 ), #4693, .F. ) ;
#32946=ORIENTED_EDGE ( 'NONE', *, *, #18244, .F. ) ;
#32955=PLANE ( 'NONE',  #2741 ) ;
#32956=AXIS2_PLACEMENT_3D ( 'NONE', #18546, #15649, #12800 ) ;
#33022=UNCERTAINTY_MEASURE_WITH_UNIT (LENGTH_MEASURE( 1.000000000000000082E-05 ), #22934, 'distance_accuracy_value', 'NONE');
#33047=EDGE_CURVE ( 'NONE', #25950, #18471, #16694, .T. ) ;
#33064=VECTOR ( 'NONE', #25679, 1000.000000000000000 ) ;
#33091=ADVANCED_FACE ( 'NONE', ( #18997 ), #2636, .T. ) ;
#33102=ORIENTED_EDGE ( 'NONE', *, *, #13892, .T. ) ;
#33213=DIRECTION ( 'NONE',  ( 0.000000000000000000, 0.5735764363510502672, -0.8191520442889889120 ) ) ;
#33292=CARTESIAN_POINT ( 'NONE',  ( 70.00000000000001421, 49.63000703270403591, 62.56502393413636298 ) ) ;
#33299=ADVANCED_FACE ( 'NONE', ( #30696 ), #25293, .T. ) ;
#33331=DIRECTION ( 'NONE',  ( -1.000000000000000000, 0.000000000000000000, 0.000000000000000000 ) ) ;
#33336=VERTEX_POINT ( 'NONE', #6025 ) ;
#33355=ORIENTED_EDGE ( 'NONE', *, *, #17819, .T. ) ;
#33425=ORIENTED_EDGE ( 'NONE', *, *, #4160, .T. ) ;
#33475=FACE_BOUND ( 'NONE', #18907, .T. ) ;
#33544=VECTOR ( 'NONE', #18056, 1000.000000000000000 ) ;
#33554=CARTESIAN_POINT ( 'NONE',  ( 115.0000000000000000, 81.48267994499606459, 30.15054357219658954 ) ) ;
#33585=CIRCLE ( 'NONE', #1975, 5.000000000000004441 ) ;
#33608=ORIENTED_EDGE ( 'NONE', *, *, #15855, .F. ) ;
#33702=ORIENTED_EDGE ( 'NONE', *, *, #24868, .F. ) ;
#33750=MANIFOLD_SOLID_BREP ( 'Cavity1', #3769 ) ;
#33799=CARTESIAN_POINT ( 'NONE',  ( 65.00000000000001421, -25.98076211353320986, 91.99999999999994316 ) ) ;
#33810=DIRECTION ( 'NONE',  ( -1.000000000000000000, 0.000000000000000000, -0.000000000000000000 ) ) ;
#33823=DIRECTION ( 'NONE',  ( 0.000000000000000000, 0.000000000000000000, -1.000000000000000000 ) ) ;
#33824=VERTEX_POINT ( 'NONE', #23554 ) ;
#33832=FILL_AREA_STYLE_COLOUR ( '', #26349 ) ;
#33932=VERTEX_POINT ( 'NONE', #22090 ) ;
#33988=CARTESIAN_POINT ( 'NONE',  ( 70.00001200000002655, -26.50436088913151167, 88.99999999999992895 ) ) ;
#34008=EDGE_LOOP ( 'NONE', ( #8980, #25653, #32555, #4592 ) ) ;
#34039=DIRECTION ( 'NONE',  ( 1.000000000000000000, 0.000000000000000000, 0.000000000000000000 ) ) ;
#34201=EDGE_LOOP ( 'NONE', ( #15492, #25699, #15662, #29277 ) ) ;
#34300=CARTESIAN_POINT ( 'NONE',  ( 65.00000000000001421, -27.93100416606587899, 81.50764321173589622 ) ) ;
#34312=DIRECTION ( 'NONE',  ( 0.000000000000000000, -0.5735764363510502672, 0.8191520442889889120 ) ) ;
#34343=CARTESIAN_POINT ( 'NONE',  ( 70.00001200000001234, -29.98076211353321341, 85.52359877559823076 ) ) ;
#34354=DIRECTION ( 'NONE',  ( -1.000000000000000000, 0.000000000000000000, 0.000000000000000000 ) ) ;
#34408=CARTESIAN_POINT ( 'NONE',  ( 63.00000000000001421, -28.31857036507964764, 80.03062855292515110 ) ) ;
#34443=VERTEX_POINT ( 'NONE', #8187 ) ;
#34486=CIRCLE ( 'NONE', #31592, 4.499999999999990230 ) ;
#34599=VERTEX_POINT ( 'NONE', #23655 ) ;
#34727=SURFACE_STYLE_USAGE ( .BOTH. , #23921 ) ;
#34779=CARTESIAN_POINT ( 'NONE',  ( 70.00001200000002655, -22.08487140685993921, 86.04699153743705153 ) ) ;
#34808=ADVANCED_FACE ( 'NONE', ( #18238 ), #15883, .F. ) ;
#34913=ORIENTED_EDGE ( 'NONE', *, *, #5358, .F. ) ;
#34927=DIRECTION ( 'NONE',  ( -1.000000000000000000, -0.000000000000000000, -0.000000000000000000 ) ) ;
#34929=ORIENTED_EDGE ( 'NONE', *, *, #19666, .T. ) ;
#34962=ORIENTED_EDGE ( 'NONE', *, *, #8556, .T. ) ;
#35094=ORIENTED_EDGE ( 'NONE', *, *, #2663, .T. ) ;
#35099=ORIENTED_EDGE ( 'NONE', *, *, #26503, .T. ) ;
#35102=AXIS2_PLACEMENT_3D ( 'NONE', #15747, #29823, #24235 ) ;
#35106=FACE_OUTER_BOUND ( 'NONE', #28526, .T. ) ;
#35131=EDGE_LOOP ( 'NONE', ( #21121, #35099, #12331, #30094 ) ) ;
#35227=DIRECTION ( 'NONE',  ( 0.000000000000000000, 0.000000000000000000, 1.000000000000000000 ) ) ;
#35262=CARTESIAN_POINT ( 'NONE',  ( 70.00000000000001421, -30.47068043442695284, 88.33026027086506815 ) ) ;
#35280=ORIENTED_EDGE ( 'NONE', *, *, #4271, .T. ) ;
#35287=ORIENTED_EDGE ( 'NONE', *, *, #27033, .T. ) ;
#35307=VERTEX_POINT ( 'NONE', #18556 ) ;
#35523=VECTOR ( 'NONE', #5598, 1000.000000000000000 ) ;
#35586=DIRECTION ( 'NONE',  ( 0.000000000000000000, -1.000000000000000000, 0.000000000000000000 ) ) ;
ENDSEC;
END-ISO-10303-21;
